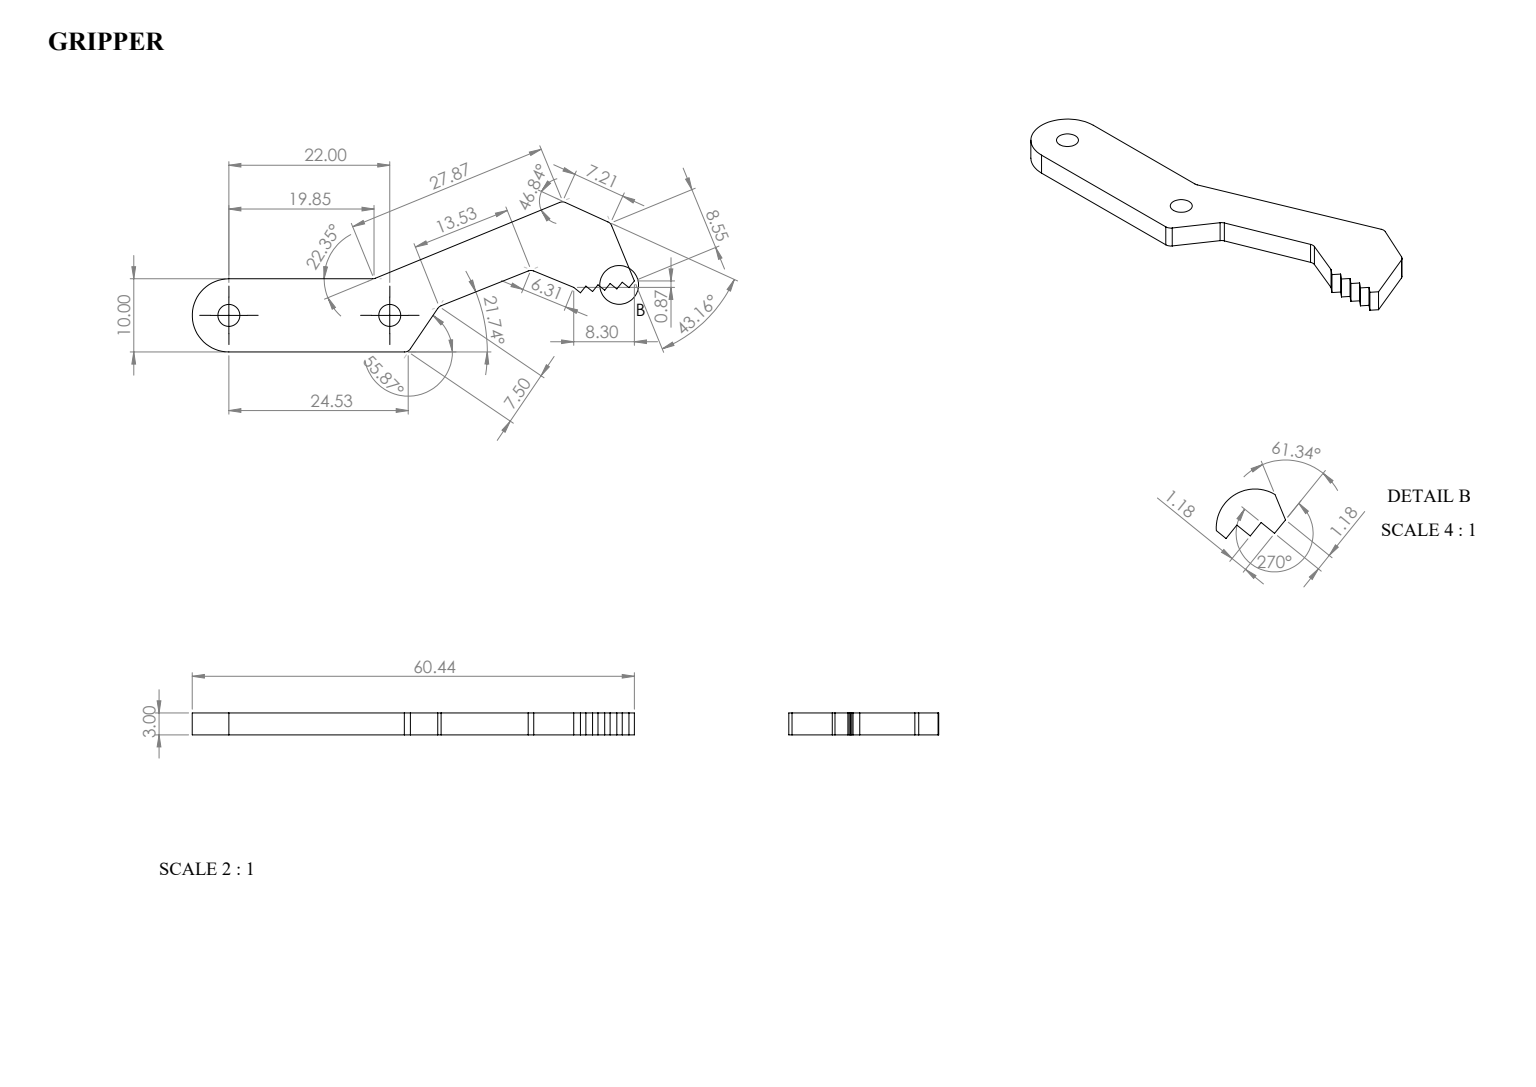
ISO-10303-21;
HEADER;
FILE_DESCRIPTION (('STEP AP214'),
    '1' );
FILE_NAME ('gripper.step',
    '2026-10-11T23:18:24',
    ( '' ),
    ( '' ),
    'SwSTEP 2.0',
    'SolidWorks 2021',
    '' );
FILE_SCHEMA (( 'AUTOMOTIVE_DESIGN' ));
ENDSEC;

DATA;
#11=PLANE ( 'NONE',  #4028 ) ;
#15=CARTESIAN_POINT ( 'NONE',  ( 45.22938609343211880, 3.000000000000000000, -15.43472716196784233 ) ) ;
#33=LINE ( 'NONE', #12635, #7280 ) ;
#53=CARTESIAN_POINT ( 'NONE',  ( 0.000000000000000000, 3.000000000000000000, 0.000000000000000000 ) ) ;
#54=CARTESIAN_POINT ( 'NONE',  ( 41.29994854050690378, 3.000000000000000000, -5.141175130212632283 ) ) ;
#66=AXIS2_PLACEMENT_3D ( 'NONE', #5412, #190, #2837 ) ;
#85=DIRECTION ( 'NONE',  ( 0.7772490812545796990, 0.000000000000000000, 0.6291930273683203900 ) ) ;
#143=DIRECTION ( 'NONE',  ( -0.6291930273683257191, 0.000000000000000000, 0.7772490812545752581 ) ) ;
#190=DIRECTION ( 'NONE',  ( -0.000000000000000000, -1.000000000000000000, -0.000000000000000000 ) ) ;
#201=DIRECTION ( 'NONE',  ( 0.6291930273683254971, 0.000000000000000000, -0.7772490812545754801 ) ) ;
#217=FACE_OUTER_BOUND ( 'NONE', #13506, .T. ) ;
#223=DIRECTION ( 'NONE',  ( -0.000000000000000000, -1.000000000000000000, -0.000000000000000000 ) ) ;
#250=ADVANCED_FACE ( 'NONE', ( #4318 ), #7479, .T. ) ;
#285=AXIS2_PLACEMENT_3D ( 'NONE', #7655, #11797, #366 ) ;
#289=DIRECTION ( 'NONE',  ( 0.7772490812545727046, 0.000000000000000000, 0.6291930273683288277 ) ) ;
#291=VERTEX_POINT ( 'NONE', #13245 ) ;
#292=ORIENTED_EDGE ( 'NONE', *, *, #12896, .T. ) ;
#295=CIRCLE ( 'NONE', #8842, 5.000000000000000000 ) ;
#344=VERTEX_POINT ( 'NONE', #5616 ) ;
#359=ORIENTED_EDGE ( 'NONE', *, *, #9429, .F. ) ;
#362=EDGE_CURVE ( 'NONE', #1968, #1088, #10282, .T. ) ;
#366=DIRECTION ( 'NONE',  ( 0.000000000000000000, 0.000000000000000000, -1.000000000000000000 ) ) ;
#372=ORIENTED_EDGE ( 'NONE', *, *, #1521, .T. ) ;
#388=EDGE_CURVE ( 'NONE', #9987, #6903, #13386, .T. ) ;
#417=ORIENTED_EDGE ( 'NONE', *, *, #1401, .T. ) ;
#424=CARTESIAN_POINT ( 'NONE',  ( 50.46378962010818015, 3.000000000000000000, -4.178819016005276943 ) ) ;
#432=EDGE_CURVE ( 'NONE', #1362, #2254, #9941, .T. ) ;
#437=DIRECTION ( 'NONE',  ( 0.6291930273683107311, 0.000000000000000000, -0.7772490812545873595 ) ) ;
#446=ORIENTED_EDGE ( 'NONE', *, *, #6514, .F. ) ;
#464=VERTEX_POINT ( 'NONE', #3179 ) ;
#465=AXIS2_PLACEMENT_3D ( 'NONE', #7088, #12335, #6953 ) ;
#488=LINE ( 'NONE', #2617, #1153 ) ;
#498=CARTESIAN_POINT ( 'NONE',  ( 0.000000000000000000, 0.000000000000000000, 5.000000000000000000 ) ) ;
#515=CARTESIAN_POINT ( 'NONE',  ( 22.00000000000000000, 0.000000000000000000, 0.000000000000000000 ) ) ;
#530=PLANE ( 'NONE',  #9767 ) ;
#532=CARTESIAN_POINT ( 'NONE',  ( 19.65244806805498357, 3.000000000000000000, -6.000000000000000000 ) ) ;
#534=CARTESIAN_POINT ( 'NONE',  ( 20.03271148078819408, 3.000000000000000000, -5.075121771833452478 ) ) ;
#572=CARTESIAN_POINT ( 'NONE',  ( 52.34174591811297717, 3.000000000000000000, -12.24483450274845531 ) ) ;
#578=VERTEX_POINT ( 'NONE', #7650 ) ;
#584=DIRECTION ( 'NONE',  ( 0.000000000000000000, 1.000000000000000000, 0.000000000000000000 ) ) ;
#587=LINE ( 'NONE', #922, #674 ) ;
#589=FACE_OUTER_BOUND ( 'NONE', #13557, .T. ) ;
#593=CARTESIAN_POINT ( 'NONE',  ( 49.72134184781355515, 0.000000000000000000, -3.261665100124877981 ) ) ;
#596=EDGE_CURVE ( 'NONE', #2976, #3318, #5708, .T. ) ;
#601=DIRECTION ( 'NONE',  ( 0.000000000000000000, 1.000000000000000000, 0.000000000000000000 ) ) ;
#610=ORIENTED_EDGE ( 'NONE', *, *, #4580, .T. ) ;
#641=VERTEX_POINT ( 'NONE', #2277 ) ;
#646=DIRECTION ( 'NONE',  ( -0.7772490812545873595, 0.000000000000000000, -0.6291930273683107311 ) ) ;
#662=AXIS2_PLACEMENT_3D ( 'NONE', #2861, #601, #2728 ) ;
#664=DIRECTION ( 'NONE',  ( 0.9248782281665489657, 0.000000000000000000, -0.3802634127332067404 ) ) ;
#666=EDGE_CURVE ( 'NONE', #1008, #7348, #6486, .T. ) ;
#674=VECTOR ( 'NONE', #7131, 1000.000000000000000 ) ;
#691=ORIENTED_EDGE ( 'NONE', *, *, #2431, .T. ) ;
#702=FACE_OUTER_BOUND ( 'NONE', #12220, .T. ) ;
#728=VECTOR ( 'NONE', #13325, 1000.000000000000000 ) ;
#731=VECTOR ( 'NONE', #11588, 1000.000000000000000 ) ;
#739=CARTESIAN_POINT ( 'NONE',  ( 53.04054522416362261, 3.000000000000000000, -3.611077387296437013 ) ) ;
#770=EDGE_CURVE ( 'NONE', #5898, #6650, #5857, .T. ) ;
#782=CIRCLE ( 'NONE', #5181, 1.500000000000000666 ) ;
#791=MECHANICAL_DESIGN_GEOMETRIC_PRESENTATION_REPRESENTATION('',(#6937),#11784);
#794=CARTESIAN_POINT ( 'NONE',  ( 20.03271148078819408, 0.000000000000000000, -5.075121771833452478 ) ) ;
#795=EDGE_CURVE ( 'NONE', #291, #13143, #3919, .T. ) ;
#799=CARTESIAN_POINT ( 'NONE',  ( 48.80418793193314997, 0.000000000000000000, -4.004112872419501201 ) ) ;
#814=DIRECTION ( 'NONE',  ( -0.4145344181384821858, 0.000000000000000000, 0.9100336346413741007 ) ) ;
#826=LINE ( 'NONE', #5339, #12157 ) ;
#830=ORIENTED_EDGE ( 'NONE', *, *, #11288, .T. ) ;
#835=( LENGTH_UNIT ( ) NAMED_UNIT ( * ) SI_UNIT ( .MILLI., .METRE. ) );
#847=ORIENTED_EDGE ( 'NONE', *, *, #2780, .F. ) ;
#860=EDGE_CURVE ( 'NONE', #10776, #641, #1589, .T. ) ;
#876=CARTESIAN_POINT ( 'NONE',  ( 29.02231267299996986, 3.000000000000000000, -1.321950885510182250 ) ) ;
#885=EDGE_CURVE ( 'NONE', #12346, #7762, #8457, .T. ) ;
#922=CARTESIAN_POINT ( 'NONE',  ( 48.80418793193314997, 3.000000000000000000, -4.004112872419501201 ) ) ;
#925=FACE_OUTER_BOUND ( 'NONE', #3987, .T. ) ;
#944=LINE ( 'NONE', #5143, #12861 ) ;
#967=ORIENTED_EDGE ( 'NONE', *, *, #13406, .T. ) ;
#977=DIRECTION ( 'NONE',  ( 0.7772490812545771455, 0.000000000000000000, 0.6291930273683233876 ) ) ;
#1007=VECTOR ( 'NONE', #3151, 1000.000000000000000 ) ;
#1008=VERTEX_POINT ( 'NONE', #7434 ) ;
#1037=DIRECTION ( 'NONE',  ( -0.7772490812545750360, 0.000000000000000000, -0.6291930273683260522 ) ) ;
#1041=EDGE_CURVE ( 'NONE', #6903, #7175, #2191, .T. ) ;
#1052=FACE_OUTER_BOUND ( 'NONE', #12922, .T. ) ;
#1074=DIRECTION ( 'NONE',  ( -0.000000000000000000, -1.000000000000000000, -0.000000000000000000 ) ) ;
#1075=ORIENTED_EDGE ( 'NONE', *, *, #12735, .T. ) ;
#1088=VERTEX_POINT ( 'NONE', #8584 ) ;
#1107=ORIENTED_EDGE ( 'NONE', *, *, #3844, .F. ) ;
#1113=ORIENTED_EDGE ( 'NONE', *, *, #9512, .F. ) ;
#1127=ORIENTED_EDGE ( 'NONE', *, *, #9053, .T. ) ;
#1150=DIRECTION ( 'NONE',  ( 0.7772490812545826966, 0.000000000000000000, 0.6291930273683166153 ) ) ;
#1153=VECTOR ( 'NONE', #7917, 1000.000000000000000 ) ;
#1160=ORIENTED_EDGE ( 'NONE', *, *, #11475, .F. ) ;
#1161=AXIS2_PLACEMENT_3D ( 'NONE', #2598, #10999, #1573 ) ;
#1187=ORIENTED_EDGE ( 'NONE', *, *, #8298, .F. ) ;
#1210=AXIS2_PLACEMENT_3D ( 'NONE', #424, #12838, #1323 ) ;
#1222=ORIENTED_EDGE ( 'NONE', *, *, #12916, .F. ) ;
#1226=DIRECTION ( 'NONE',  ( 0.6291930273683290498, 0.000000000000000000, -0.7772490812545727046 ) ) ;
#1244=CARTESIAN_POINT ( 'NONE',  ( 23.99887587215152607, 3.000000000000000000, 4.000000000000000000 ) ) ;
#1250=CARTESIAN_POINT ( 'NONE',  ( 19.65244806805498001, 3.000000000000000000, -5.000000000000000000 ) ) ;
#1264=ORIENTED_EDGE ( 'NONE', *, *, #2886, .T. ) ;
#1265=ORIENTED_EDGE ( 'NONE', *, *, #666, .F. ) ;
#1281=LINE ( 'NONE', #10781, #3594 ) ;
#1294=ORIENTED_EDGE ( 'NONE', *, *, #11288, .F. ) ;
#1297=ADVANCED_FACE ( 'NONE', ( #5972 ), #12048, .F. ) ;
#1311=ORIENTED_EDGE ( 'NONE', *, *, #885, .F. ) ;
#1313=ORIENTED_EDGE ( 'NONE', *, *, #10118, .T. ) ;
#1323=DIRECTION ( 'NONE',  ( -0.7772490812545771455, 0.000000000000000000, -0.6291930273683233876 ) ) ;
#1325=DIRECTION ( 'NONE',  ( -0.9288742131985401329, 0.000000000000000000, 0.3703953240185315909 ) ) ;
#1342=EDGE_CURVE ( 'NONE', #7762, #9987, #8243, .T. ) ;
#1348=DIRECTION ( 'NONE',  ( 0.5610724890695777400, 0.000000000000000000, -0.8277666712360848278 ) ) ;
#1352=DIRECTION ( 'NONE',  ( 0.6291930273683254971, 0.000000000000000000, -0.7772490812545754801 ) ) ;
#1362=VERTEX_POINT ( 'NONE', #4171 ) ;
#1373=DIRECTION ( 'NONE',  ( 0.000000000000000000, 1.000000000000000000, 0.000000000000000000 ) ) ;
#1383=VERTEX_POINT ( 'NONE', #6116 ) ;
#1401=EDGE_CURVE ( 'NONE', #12205, #5887, #5126, .T. ) ;
#1404=VECTOR ( 'NONE', #9043, 1000.000000000000000 ) ;
#1411=CARTESIAN_POINT ( 'NONE',  ( 0.000000000000000000, 3.000000000000000000, 0.000000000000000000 ) ) ;
#1419=VERTEX_POINT ( 'NONE', #4785 ) ;
#1443=AXIS2_PLACEMENT_3D ( 'NONE', #11916, #10885, #1450 ) ;
#1445=EDGE_CURVE ( 'NONE', #11616, #8766, #4718, .T. ) ;
#1450=DIRECTION ( 'NONE',  ( 0.000000000000000000, 0.000000000000000000, -1.000000000000000000 ) ) ;
#1475=CARTESIAN_POINT ( 'NONE',  ( 47.14458624375820506, 0.000000000000000000, -3.829406728833672613 ) ) ;
#1511=CARTESIAN_POINT ( 'NONE',  ( 29.39270799701850123, 3.000000000000000000, -0.3930766723116408401 ) ) ;
#1521=EDGE_CURVE ( 'NONE', #3318, #464, #2714, .T. ) ;
#1564=CARTESIAN_POINT ( 'NONE',  ( 22.00000000000000000, 3.000000000000000000, -1.500000000000000666 ) ) ;
#1569=EDGE_CURVE ( 'NONE', #5437, #5898, #5276, .T. ) ;
#1573=DIRECTION ( 'NONE',  ( -1.000000000000000000, 0.000000000000000000, -0.000000000000000000 ) ) ;
#1589=LINE ( 'NONE', #3857, #4670 ) ;
#1592=VERTEX_POINT ( 'NONE', #12597 ) ;
#1605=PRODUCT_DEFINITION ( 'UNKNOWN', '', #8267, #12345 ) ;
#1606=FACE_OUTER_BOUND ( 'NONE', #1630, .T. ) ;
#1628=EDGE_LOOP ( 'NONE', ( #967, #8471, #2768, #4879 ) ) ;
#1630=EDGE_LOOP ( 'NONE', ( #9979, #6504, #3840, #12459, #9427, #11054, #12260, #11882, #1794, #1294, #6593, #5923, #12223, #9618, #6732, #1311, #5467, #13454, #10169, #1160, #8458, #5363, #5414, #7618, #8830, #3725, #12842 ) ) ;
#1636=CARTESIAN_POINT ( 'NONE',  ( 45.60964950616533287, 0.000000000000000000, -14.50984893380129392 ) ) ;
#1637=FACE_OUTER_BOUND ( 'NONE', #7799, .T. ) ;
#1665=CARTESIAN_POINT ( 'NONE',  ( 54.70014691233865989, 3.000000000000000000, -3.785783530882224746 ) ) ;
#1671=DIRECTION ( 'NONE',  ( -0.7772490812546181127, 0.000000000000000000, -0.6291930273682727615 ) ) ;
#1683=ORIENTED_EDGE ( 'NONE', *, *, #770, .T. ) ;
#1724=DIRECTION ( 'NONE',  ( 0.000000000000000000, 0.000000000000000000, -1.000000000000000000 ) ) ;
#1733=EDGE_CURVE ( 'NONE', #8766, #12346, #10724, .T. ) ;
#1738=FACE_OUTER_BOUND ( 'NONE', #5719, .T. ) ;
#1770=VECTOR ( 'NONE', #4286, 1000.000000000000000 ) ;
#1773=EDGE_CURVE ( 'NONE', #3986, #6650, #1281, .T. ) ;
#1780=CIRCLE ( 'NONE', #9471, 1.000000000000000888 ) ;
#1781=ORIENTED_EDGE ( 'NONE', *, *, #2886, .F. ) ;
#1788=EDGE_CURVE ( 'NONE', #2335, #10776, #7481, .T. ) ;
#1794=ORIENTED_EDGE ( 'NONE', *, *, #13063, .F. ) ;
#1804=CARTESIAN_POINT ( 'NONE',  ( 22.00000000000000000, 3.000000000000000000, -1.500000000000000666 ) ) ;
#1840=DIRECTION ( 'NONE',  ( 0.000000000000000000, 0.000000000000000000, -1.000000000000000000 ) ) ;
#1850=VECTOR ( 'NONE', #1150, 1000.000000000000227 ) ;
#1863=DIRECTION ( 'NONE',  ( -0.000000000000000000, -1.000000000000000000, -0.000000000000000000 ) ) ;
#1867=ORIENTED_EDGE ( 'NONE', *, *, #432, .T. ) ;
#1877=SURFACE_SIDE_STYLE ('',( #11233 ) ) ;
#1901=EDGE_CURVE ( 'NONE', #6718, #12346, #8914, .T. ) ;
#1918=CYLINDRICAL_SURFACE ( 'NONE', #5087, 1.000000000000000888 ) ;
#1942=DIRECTION ( 'NONE',  ( -0.000000000000000000, -1.000000000000000000, -0.000000000000000000 ) ) ;
#1962=ORIENTED_EDGE ( 'NONE', *, *, #388, .T. ) ;
#1968=VERTEX_POINT ( 'NONE', #6164 ) ;
#1973=CARTESIAN_POINT ( 'NONE',  ( 55.44259468463320673, 3.000000000000000000, -4.702937446762657459 ) ) ;
#1996=ORIENTED_EDGE ( 'NONE', *, *, #12521, .F. ) ;
#2009=LINE ( 'NONE', #6271, #5183 ) ;
#2019=DIRECTION ( 'NONE',  ( 0.000000000000000000, 0.000000000000000000, 1.000000000000000000 ) ) ;
#2026=AXIS2_PLACEMENT_3D ( 'NONE', #8392, #1373, #7643 ) ;
#2035=VECTOR ( 'NONE', #4236, 1000.000000000000000 ) ;
#2052=CARTESIAN_POINT ( 'NONE',  ( 24.82664254338761722, 3.000000000000000000, 4.561072489069574409 ) ) ;
#2058=DIRECTION ( 'NONE',  ( -0.000000000000000000, -1.000000000000000000, -0.000000000000000000 ) ) ;
#2061=DIRECTION ( 'NONE',  ( -0.000000000000000000, -1.000000000000000000, -0.000000000000000000 ) ) ;
#2082=VERTEX_POINT ( 'NONE', #11267 ) ;
#2085=DIRECTION ( 'NONE',  ( 0.000000000000000000, 0.000000000000000000, -1.000000000000000000 ) ) ;
#2088=DIRECTION ( 'NONE',  ( 0.000000000000000000, 0.000000000000000000, -1.000000000000000000 ) ) ;
#2099=VERTEX_POINT ( 'NONE', #10241 ) ;
#2102=ORIENTED_EDGE ( 'NONE', *, *, #8983, .T. ) ;
#2144=ORIENTED_EDGE ( 'NONE', *, *, #7522, .T. ) ;
#2169=DIRECTION ( 'NONE',  ( 0.6291930273683260522, 0.000000000000000000, -0.7772490812545749250 ) ) ;
#2171=PLANE ( 'NONE',  #12135 ) ;
#2187=LINE ( 'NONE', #11973, #6238 ) ;
#2191=LINE ( 'NONE', #13571, #2255 ) ;
#2203=ORIENTED_EDGE ( 'NONE', *, *, #4595, .T. ) ;
#2216=CARTESIAN_POINT ( 'NONE',  ( 53.78299299645824050, 3.000000000000000000, -4.528231303176834643 ) ) ;
#2239=VERTEX_POINT ( 'NONE', #10842 ) ;
#2246=CIRCLE ( 'NONE', #285, 1.000000000000000000 ) ;
#2247=AXIS2_PLACEMENT_3D ( 'NONE', #12014, #2569, #13172 ) ;
#2248=CARTESIAN_POINT ( 'NONE',  ( 47.14458624375820506, 3.000000000000000000, -3.829406728833672613 ) ) ;
#2254=VERTEX_POINT ( 'NONE', #7933 ) ;
#2255=VECTOR ( 'NONE', #6389, 1000.000000000000000 ) ;
#2268=VECTOR ( 'NONE', #13335, 1000.000000000000000 ) ;
#2277=CARTESIAN_POINT ( 'NONE',  ( 48.80418793193314997, 0.000000000000000000, -4.004112872419501201 ) ) ;
#2278=EDGE_CURVE ( 'NONE', #2254, #7268, #10593, .T. ) ;
#2293=CARTESIAN_POINT ( 'NONE',  ( 0.000000000000000000, 3.000000000000000000, 5.000000000000000000 ) ) ;
#2299=ORIENTED_EDGE ( 'NONE', *, *, #795, .T. ) ;
#2312=PLANE ( 'NONE',  #8209 ) ;
#2335=VERTEX_POINT ( 'NONE', #1475 ) ;
#2336=PRODUCT_CONTEXT ( 'NONE', #3509, 'mechanical' ) ;
#2385=CARTESIAN_POINT ( 'NONE',  ( 52.12339130828321032, 0.000000000000000000, -4.353525159591052685 ) ) ;
#2388=EDGE_CURVE ( 'NONE', #11595, #10663, #6143, .T. ) ;
#2392=CARTESIAN_POINT ( 'NONE',  ( 41.67875868938293138, 0.000000000000000000, -6.066649533482935119 ) ) ;
#2395=ORIENTED_EDGE ( 'NONE', *, *, #8983, .F. ) ;
#2431=EDGE_CURVE ( 'NONE', #4566, #7781, #13590, .T. ) ;
#2458=DIRECTION ( 'NONE',  ( 0.9254744032703045020, 0.000000000000000000, 0.3788101488760216018 ) ) ;
#2476=CYLINDRICAL_SURFACE ( 'NONE', #4736, 1.000000000000000444 ) ;
#2505=ORIENTED_EDGE ( 'NONE', *, *, #13043, .F. ) ;
#2518=CIRCLE ( 'NONE', #8237, 1.500000000000000222 ) ;
#2520=VECTOR ( 'NONE', #3875, 1000.000000000000000 ) ;
#2524=DIRECTION ( 'NONE',  ( 0.000000000000000000, 0.000000000000000000, 1.000000000000000000 ) ) ;
#2531=DIRECTION ( 'NONE',  ( -0.000000000000000000, -1.000000000000000000, -0.000000000000000000 ) ) ;
#2533=EDGE_LOOP ( 'NONE', ( #3440, #12296, #7097, #7171 ) ) ;
#2551=LINE ( 'NONE', #8373, #7050 ) ;
#2568=EDGE_LOOP ( 'NONE', ( #11980, #11539, #3859, #1127 ) ) ;
#2569=DIRECTION ( 'NONE',  ( 0.000000000000000000, -1.000000000000000000, 0.000000000000000000 ) ) ;
#2575=PLANE ( 'NONE',  #10618 ) ;
#2598=CARTESIAN_POINT ( 'NONE',  ( 0.000000000000000000, 3.000000000000000000, 5.000000000000000000 ) ) ;
#2617=CARTESIAN_POINT ( 'NONE',  ( 45.60964950616533287, 3.000000000000000000, -15.50984893380129392 ) ) ;
#2622=LINE ( 'NONE', #3865, #12146 ) ;
#2649=DIRECTION ( 'NONE',  ( 0.000000000000000000, 0.000000000000000000, -1.000000000000000000 ) ) ;
#2691=DIRECTION ( 'NONE',  ( -0.9100336346413742117, -0.000000000000000000, -0.4145344181384821858 ) ) ;
#2694=FACE_BOUND ( 'NONE', #2698, .T. ) ;
#2698=EDGE_LOOP ( 'NONE', ( #8476, #417 ) ) ;
#2700=ORIENTED_EDGE ( 'NONE', *, *, #7210, .T. ) ;
#2714=LINE ( 'NONE', #11189, #4255 ) ;
#2728=DIRECTION ( 'NONE',  ( 0.000000000000000000, 0.000000000000000000, 1.000000000000000000 ) ) ;
#2751=CARTESIAN_POINT ( 'NONE',  ( 53.04054522416362261, 0.000000000000000000, -3.611077387296437013 ) ) ;
#2759=EDGE_LOOP ( 'NONE', ( #4791, #11244, #3057, #10602 ) ) ;
#2768=ORIENTED_EDGE ( 'NONE', *, *, #4568, .F. ) ;
#2780=EDGE_CURVE ( 'NONE', #13316, #10663, #7108, .T. ) ;
#2784=CARTESIAN_POINT ( 'NONE',  ( 29.02231267299996986, 3.000000000000000000, -1.321950885510182250 ) ) ;
#2787=ORIENTED_EDGE ( 'NONE', *, *, #9935, .F. ) ;
#2792=DIRECTION ( 'NONE',  ( 0.000000000000000000, 1.000000000000000000, -0.000000000000000000 ) ) ;
#2803=EDGE_LOOP ( 'NONE', ( #5343, #13058, #2787, #6487 ) ) ;
#2804=ORIENTED_EDGE ( 'NONE', *, *, #12721, .F. ) ;
#2811=DIRECTION ( 'NONE',  ( 0.000000000000000000, 1.000000000000000000, -0.000000000000000000 ) ) ;
#2826=CARTESIAN_POINT ( 'NONE',  ( 51.41686768994642165, 3.000000000000000000, -11.86457109001525545 ) ) ;
#2837=DIRECTION ( 'NONE',  ( 0.000000000000000000, 0.000000000000000000, -1.000000000000000000 ) ) ;
#2849=DIRECTION ( 'NONE',  ( 0.6291930273682743158, 0.000000000000000000, -0.7772490812546168915 ) ) ;
#2861=CARTESIAN_POINT ( 'NONE',  ( 22.00000000000000000, 3.000000000000000000, 0.000000000000000000 ) ) ;
#2864=PLANE ( 'NONE',  #6038 ) ;
#2865=CARTESIAN_POINT ( 'NONE',  ( 24.82664254338761722, 3.000000000000000000, 4.561072489069574409 ) ) ;
#2880=CIRCLE ( 'NONE', #10802, 1.500000000000000666 ) ;
#2882=AXIS2_PLACEMENT_3D ( 'NONE', #2248, #1226, #11762 ) ;
#2886=EDGE_CURVE ( 'NONE', #2239, #2099, #3058, .T. ) ;
#2892=EDGE_CURVE ( 'NONE', #6179, #5887, #11232, .T. ) ;
#2913=VECTOR ( 'NONE', #11160, 1000.000000000000000 ) ;
#2923=CARTESIAN_POINT ( 'NONE',  ( 52.12339130828321032, 3.000000000000000000, -4.353525159591052685 ) ) ;
#2938=DIRECTION ( 'NONE',  ( 0.000000000000000000, 0.000000000000000000, -1.000000000000000000 ) ) ;
#2970=CARTESIAN_POINT ( 'NONE',  ( 53.04054522416362261, 3.000000000000000000, -3.611077387296437013 ) ) ;
#2976=VERTEX_POINT ( 'NONE', #3286 ) ;
#3050=DIRECTION ( 'NONE',  ( -0.000000000000000000, -1.000000000000000000, -0.000000000000000000 ) ) ;
#3053=ORIENTED_EDGE ( 'NONE', *, *, #3579, .T. ) ;
#3055=ORIENTED_EDGE ( 'NONE', *, *, #596, .T. ) ;
#3057=ORIENTED_EDGE ( 'NONE', *, *, #1569, .F. ) ;
#3058=CIRCLE ( 'NONE', #8763, 0.9999999999999991118 ) ;
#3079=DIRECTION ( 'NONE',  ( 0.000000000000000000, 0.000000000000000000, 1.000000000000000000 ) ) ;
#3091=VECTOR ( 'NONE', #3849, 1000.000000000000114 ) ;
#3101=EDGE_LOOP ( 'NONE', ( #12387, #11429 ) ) ;
#3102=ORIENTED_EDGE ( 'NONE', *, *, #6600, .T. ) ;
#3120=ADVANCED_FACE ( 'NONE', ( #3564, #11005, #6676 ), #12050, .F. ) ;
#3129=CARTESIAN_POINT ( 'NONE',  ( 0.000000000000000000, 3.000000000000000000, -1.500000000000000222 ) ) ;
#3151=DIRECTION ( 'NONE',  ( -0.000000000000000000, -1.000000000000000000, -0.000000000000000000 ) ) ;
#3173=PLANE ( 'NONE',  #6883 ) ;
#3179=CARTESIAN_POINT ( 'NONE',  ( 48.80418793193314997, 3.000000000000000000, -4.004112872419501201 ) ) ;
#3217=EDGE_CURVE ( 'NONE', #5437, #3986, #13288, .T. ) ;
#3222=ORIENTED_EDGE ( 'NONE', *, *, #795, .F. ) ;
#3239=ORIENTED_EDGE ( 'NONE', *, *, #1342, .T. ) ;
#3286=CARTESIAN_POINT ( 'NONE',  ( 47.14458624375820506, 3.000000000000000000, -3.829406728833672613 ) ) ;
#3293=CARTESIAN_POINT ( 'NONE',  ( 41.67875868938293138, 0.000000000000000000, -6.066649533482935119 ) ) ;
#3318=VERTEX_POINT ( 'NONE', #4115 ) ;
#3333=ORIENTED_EDGE ( 'NONE', *, *, #13043, .T. ) ;
#3365=AXIS2_PLACEMENT_3D ( 'NONE', #7869, #9118, #12090 ) ;
#3369=DIRECTION ( 'NONE',  ( -0.000000000000000000, -1.000000000000000000, -0.000000000000000000 ) ) ;
#3381=DIRECTION ( 'NONE',  ( 0.000000000000000000, 0.000000000000000000, 1.000000000000000000 ) ) ;
#3429=DIRECTION ( 'NONE',  ( 0.000000000000000000, 0.000000000000000000, -1.000000000000000000 ) ) ;
#3440=ORIENTED_EDGE ( 'NONE', *, *, #1788, .T. ) ;
#3447=LINE ( 'NONE', #2216, #8622 ) ;
#3453=FACE_OUTER_BOUND ( 'NONE', #2568, .T. ) ;
#3473=EDGE_CURVE ( 'NONE', #10535, #2976, #2551, .T. ) ;
#3509=APPLICATION_CONTEXT ( 'automotive_design' ) ;
#3546=LINE ( 'NONE', #6657, #12791 ) ;
#3564=FACE_OUTER_BOUND ( 'NONE', #5744, .T. ) ;
#3579=EDGE_CURVE ( 'NONE', #2082, #13415, #3666, .T. ) ;
#3592=PLANE ( 'NONE',  #2247 ) ;
#3594=VECTOR ( 'NONE', #1348, 1000.000000000000000 ) ;
#3641=ORIENTED_EDGE ( 'NONE', *, *, #13521, .T. ) ;
#3656=FACE_BOUND ( 'NONE', #5012, .T. ) ;
#3657=EDGE_CURVE ( 'NONE', #12875, #1362, #8214, .T. ) ;
#3660=ORIENTED_EDGE ( 'NONE', *, *, #6391, .T. ) ;
#3666=LINE ( 'NONE', #4841, #5489 ) ;
#3671=DIRECTION ( 'NONE',  ( 0.9288742131985401329, 0.000000000000000000, -0.3703953240185316464 ) ) ;
#3679=CARTESIAN_POINT ( 'NONE',  ( 41.29994854050690378, 3.000000000000000000, -5.141175130212632283 ) ) ;
#3680=CARTESIAN_POINT ( 'NONE',  ( 20.03271148078819408, 3.000000000000000000, -5.075121771833452478 ) ) ;
#3709=EDGE_LOOP ( 'NONE', ( #13077, #1222, #9830, #691 ) ) ;
#3712=( NAMED_UNIT ( * ) PLANE_ANGLE_UNIT ( ) SI_UNIT ( $, .RADIAN. ) );
#3725=ORIENTED_EDGE ( 'NONE', *, *, #432, .F. ) ;
#3734=DIRECTION ( 'NONE',  ( -0.7772490812545826966, 0.000000000000000000, -0.6291930273683166153 ) ) ;
#3772=DIRECTION ( 'NONE',  ( -0.000000000000000000, -1.000000000000000000, 0.000000000000000000 ) ) ;
#3777=UNCERTAINTY_MEASURE_WITH_UNIT (LENGTH_MEASURE( 1.000000000000000082E-05 ), #12389, 'distance_accuracy_value', 'NONE');
#3786=CARTESIAN_POINT ( 'NONE',  ( 51.38094353598858532, 3.000000000000000000, -3.436371243710653722 ) ) ;
#3787=PLANE ( 'NONE',  #10165 ) ;
#3789=VECTOR ( 'NONE', #6193, 1000.000000000000227 ) ;
#3840=ORIENTED_EDGE ( 'NONE', *, *, #5536, .F. ) ;
#3844=EDGE_CURVE ( 'NONE', #1008, #1968, #11860, .T. ) ;
#3849=DIRECTION ( 'NONE',  ( 0.9288742131985401329, 0.000000000000000000, -0.3703953240185316464 ) ) ;
#3857=CARTESIAN_POINT ( 'NONE',  ( 48.06174015963858892, 0.000000000000000000, -3.086958956539055166 ) ) ;
#3859=ORIENTED_EDGE ( 'NONE', *, *, #6600, .F. ) ;
#3865=CARTESIAN_POINT ( 'NONE',  ( 46.02418392430381999, 3.000000000000000000, -15.41988256844266658 ) ) ;
#3875=DIRECTION ( 'NONE',  ( -0.000000000000000000, -1.000000000000000000, -0.000000000000000000 ) ) ;
#3897=DIRECTION ( 'NONE',  ( -0.000000000000000000, -1.000000000000000000, -0.000000000000000000 ) ) ;
#3899=EDGE_CURVE ( 'NONE', #291, #9987, #33, .T. ) ;
#3903=ORIENTED_EDGE ( 'NONE', *, *, #7030, .T. ) ;
#3919=LINE ( 'NONE', #1665, #5113 ) ;
#3933=CARTESIAN_POINT ( 'NONE',  ( 54.70014691233865989, 0.000000000000000000, -3.785783530882224746 ) ) ;
#3963=VECTOR ( 'NONE', #85, 1000.000000000000000 ) ;
#3964=DIRECTION ( 'NONE',  ( -0.000000000000000000, -1.000000000000000000, -0.000000000000000000 ) ) ;
#3971=AXIS2_PLACEMENT_3D ( 'NONE', #11570, #9560, #5477 ) ;
#3977=FACE_OUTER_BOUND ( 'NONE', #3709, .T. ) ;
#3980=AXIS2_PLACEMENT_3D ( 'NONE', #54, #8234, #2938 ) ;
#3983=CIRCLE ( 'NONE', #6188, 1.500000000000000222 ) ;
#3986=VERTEX_POINT ( 'NONE', #12961 ) ;
#3987=EDGE_LOOP ( 'NONE', ( #11228, #3641, #5133, #6699 ) ) ;
#3991=CIRCLE ( 'NONE', #11480, 1.500000000000000222 ) ;
#4023=ORIENTED_EDGE ( 'NONE', *, *, #8102, .F. ) ;
#4027=ORIENTED_EDGE ( 'NONE', *, *, #5513, .T. ) ;
#4028=AXIS2_PLACEMENT_3D ( 'NONE', #2970, #1037, #7035 ) ;
#4053=AXIS2_PLACEMENT_3D ( 'NONE', #12272, #2811, #4605 ) ;
#4057=CARTESIAN_POINT ( 'NONE',  ( 29.02231267299996986, 3.000000000000000000, -1.321950885510182250 ) ) ;
#4059=UNCERTAINTY_MEASURE_WITH_UNIT (LENGTH_MEASURE( 1.000000000000000082E-05 ), #5864, 'distance_accuracy_value', 'NONE');
#4080=EDGE_LOOP ( 'NONE', ( #12049, #4926, #1107, #10377 ) ) ;
#4093=LINE ( 'NONE', #2923, #7517 ) ;
#4106=LINE ( 'NONE', #3129, #9476 ) ;
#4115=CARTESIAN_POINT ( 'NONE',  ( 48.06174015963858892, 3.000000000000000000, -3.086958956539055166 ) ) ;
#4136=CARTESIAN_POINT ( 'NONE',  ( 22.00000000000000000, 0.000000000000000000, 1.500000000000000666 ) ) ;
#4144=EDGE_CURVE ( 'NONE', #11098, #578, #1780, .T. ) ;
#4171=CARTESIAN_POINT ( 'NONE',  ( 40.92955321648837241, 0.000000000000000000, -6.070049343411170639 ) ) ;
#4172=EDGE_CURVE ( 'NONE', #464, #4566, #7379, .T. ) ;
#4187=ORIENTED_EDGE ( 'NONE', *, *, #12187, .T. ) ;
#4214=VECTOR ( 'NONE', #10335, 1000.000000000000227 ) ;
#4233=DIRECTION ( 'NONE',  ( 0.000000000000000000, 1.000000000000000000, 0.000000000000000000 ) ) ;
#4234=FACE_OUTER_BOUND ( 'NONE', #5627, .T. ) ;
#4236=DIRECTION ( 'NONE',  ( -0.000000000000000000, -1.000000000000000000, -0.000000000000000000 ) ) ;
#4255=VECTOR ( 'NONE', #2849, 1000.000000000000000 ) ;
#4260=ORIENTED_EDGE ( 'NONE', *, *, #4172, .F. ) ;
#4278=MECHANICAL_DESIGN_GEOMETRIC_PRESENTATION_REPRESENTATION('',(#12869),#7584);
#4286=DIRECTION ( 'NONE',  ( -1.000000000000000000, -0.000000000000000000, -0.000000000000000000 ) ) ;
#4318=FACE_OUTER_BOUND ( 'NONE', #8137, .T. ) ;
#4354=DIRECTION ( 'NONE',  ( 0.000000000000000000, 1.000000000000000000, 0.000000000000000000 ) ) ;
#4383=DIRECTION ( 'NONE',  ( 0.000000000000000000, 1.000000000000000000, 0.000000000000000000 ) ) ;
#4387=CARTESIAN_POINT ( 'NONE',  ( 47.14458624375820506, 3.000000000000000000, -3.829406728833672613 ) ) ;
#4403=AXIS2_PLACEMENT_3D ( 'NONE', #11454, #8084, #10427 ) ;
#4424=EDGE_LOOP ( 'NONE', ( #7431, #7570, #10921, #12591 ) ) ;
#4430=ADVANCED_FACE ( 'NONE', ( #3977 ), #11215, .F. ) ;
#4460=ORIENTED_EDGE ( 'NONE', *, *, #3473, .T. ) ;
#4501=ADVANCED_FACE ( 'NONE', ( #5979 ), #5281, .F. ) ;
#4521=DIRECTION ( 'NONE',  ( 0.7772490812545727046, 0.000000000000000000, 0.6291930273683288277 ) ) ;
#4566=VERTEX_POINT ( 'NONE', #11490 ) ;
#4568=EDGE_CURVE ( 'NONE', #5777, #9675, #11903, .T. ) ;
#4580=EDGE_CURVE ( 'NONE', #13415, #7348, #9904, .T. ) ;
#4595=EDGE_CURVE ( 'NONE', #7175, #10532, #5298, .T. ) ;
#4603=DIRECTION ( 'NONE',  ( 0.000000000000000000, -1.000000000000000000, 0.000000000000000000 ) ) ;
#4605=DIRECTION ( 'NONE',  ( 0.000000000000000000, 0.000000000000000000, -1.000000000000000000 ) ) ;
#4607=CYLINDRICAL_SURFACE ( 'NONE', #1443, 0.9999999999999991118 ) ;
#4652=CYLINDRICAL_SURFACE ( 'NONE', #7572, 1.000000000000000888 ) ;
#4670=VECTOR ( 'NONE', #5919, 1000.000000000000000 ) ;
#4717=DIRECTION ( 'NONE',  ( 0.000000000000000000, 1.000000000000000000, 0.000000000000000000 ) ) ;
#4718=LINE ( 'NONE', #10232, #1404 ) ;
#4735=CARTESIAN_POINT ( 'NONE',  ( 46.02418392430381999, 0.000000000000000000, -15.41988256844266836 ) ) ;
#4736=AXIS2_PLACEMENT_3D ( 'NONE', #1244, #3369, #10745 ) ;
#4739=ORIENTED_EDGE ( 'NONE', *, *, #13063, .T. ) ;
#4743=EDGE_CURVE ( 'NONE', #4566, #1383, #3546, .T. ) ;
#4779=DIRECTION ( 'NONE',  ( 0.000000000000000000, 0.000000000000000000, 1.000000000000000000 ) ) ;
#4785=CARTESIAN_POINT ( 'NONE',  ( 29.02231267299996986, 0.000000000000000000, -1.321950885510182250 ) ) ;
#4789=EDGE_CURVE ( 'NONE', #13316, #11616, #4859, .T. ) ;
#4791=ORIENTED_EDGE ( 'NONE', *, *, #1773, .T. ) ;
#4798=DIRECTION ( 'NONE',  ( 0.000000000000000000, 1.000000000000000000, 0.000000000000000000 ) ) ;
#4800=DIRECTION ( 'NONE',  ( -0.000000000000000000, -1.000000000000000000, -0.000000000000000000 ) ) ;
#4810=CARTESIAN_POINT ( 'NONE',  ( 29.39270799701850123, 0.000000000000000000, -0.3930766723116408401 ) ) ;
#4817=EDGE_CURVE ( 'NONE', #6179, #12863, #8590, .T. ) ;
#4841=CARTESIAN_POINT ( 'NONE',  ( 20.03271148078819408, 3.000000000000000000, -5.075121771833452478 ) ) ;
#4859=LINE ( 'NONE', #6935, #6806 ) ;
#4860=FACE_OUTER_BOUND ( 'NONE', #2803, .T. ) ;
#4879=ORIENTED_EDGE ( 'NONE', *, *, #6391, .F. ) ;
#4907=EDGE_LOOP ( 'NONE', ( #7267, #10315, #4739, #12364 ) ) ;
#4926=ORIENTED_EDGE ( 'NONE', *, *, #362, .F. ) ;
#4933=VECTOR ( 'NONE', #7075, 1000.000000000000000 ) ;
#4990=CARTESIAN_POINT ( 'NONE',  ( 53.04054522416362261, 3.000000000000000000, -3.611077387296437013 ) ) ;
#5005=EDGE_CURVE ( 'NONE', #13346, #11587, #3983, .T. ) ;
#5008=PLANE ( 'NONE',  #7556 ) ;
#5012=EDGE_LOOP ( 'NONE', ( #10920, #8741 ) ) ;
#5029=FACE_OUTER_BOUND ( 'NONE', #7031, .T. ) ;
#5059=ORIENTED_EDGE ( 'NONE', *, *, #9844, .T. ) ;
#5071=LINE ( 'NONE', #5966, #4933 ) ;
#5072=DIRECTION ( 'NONE',  ( -0.000000000000000000, -1.000000000000000000, -0.000000000000000000 ) ) ;
#5087=AXIS2_PLACEMENT_3D ( 'NONE', #6170, #5142, #11552 ) ;
#5113=VECTOR ( 'NONE', #11227, 1000.000000000000000 ) ;
#5120=DIRECTION ( 'NONE',  ( -0.000000000000000000, -1.000000000000000000, -0.000000000000000000 ) ) ;
#5126=CIRCLE ( 'NONE', #12617, 1.500000000000000666 ) ;
#5129=VECTOR ( 'NONE', #9308, 1000.000000000000000 ) ;
#5133=ORIENTED_EDGE ( 'NONE', *, *, #2892, .T. ) ;
#5142=DIRECTION ( 'NONE',  ( -0.000000000000000000, -1.000000000000000000, -0.000000000000000000 ) ) ;
#5143=CARTESIAN_POINT ( 'NONE',  ( 50.46378962010818015, 3.000000000000000000, -4.178819016005276943 ) ) ;
#5158=CIRCLE ( 'NONE', #11095, 1.000000000000000000 ) ;
#5161=FACE_OUTER_BOUND ( 'NONE', #11995, .T. ) ;
#5165=EDGE_LOOP ( 'NONE', ( #3239, #10236, #1113, #2102 ) ) ;
#5181=AXIS2_PLACEMENT_3D ( 'NONE', #8405, #4354, #2019 ) ;
#5182=CARTESIAN_POINT ( 'NONE',  ( 0.000000000000000000, 3.000000000000000000, 5.000000000000000000 ) ) ;
#5183=VECTOR ( 'NONE', #977, 1000.000000000000227 ) ;
#5196=DIRECTION ( 'NONE',  ( 0.000000000000000000, 0.000000000000000000, -1.000000000000000000 ) ) ;
#5214=CARTESIAN_POINT ( 'NONE',  ( 53.78299299645824050, 0.000000000000000000, -4.528231303176834643 ) ) ;
#5223=CARTESIAN_POINT ( 'NONE',  ( 23.99887587215152251, 3.000000000000000000, 5.000000000000000888 ) ) ;
#5240=EDGE_CURVE ( 'NONE', #7348, #1088, #6095, .T. ) ;
#5269=DIRECTION ( 'NONE',  ( -0.000000000000000000, -1.000000000000000000, -0.000000000000000000 ) ) ;
#5276=LINE ( 'NONE', #2052, #9544 ) ;
#5281=PLANE ( 'NONE',  #2882 ) ;
#5298=CIRCLE ( 'NONE', #3971, 0.9999999999999991118 ) ;
#5317=CARTESIAN_POINT ( 'NONE',  ( 51.83140210808490167, 0.000000000000000000, -12.77460472465662988 ) ) ;
#5339=CARTESIAN_POINT ( 'NONE',  ( 41.67875868938293138, 3.000000000000000000, -6.066649533482935119 ) ) ;
#5343=ORIENTED_EDGE ( 'NONE', *, *, #7094, .T. ) ;
#5344=ADVANCED_FACE ( 'NONE', ( #925 ), #7506, .F. ) ;
#5352=DIRECTION ( 'NONE',  ( 0.000000000000000000, 0.000000000000000000, 1.000000000000000000 ) ) ;
#5363=ORIENTED_EDGE ( 'NONE', *, *, #860, .F. ) ;
#5396=EDGE_LOOP ( 'NONE', ( #1996, #359, #9297, #1867 ) ) ;
#5403=ADVANCED_FACE ( 'NONE', ( #6913 ), #5668, .F. ) ;
#5412=CARTESIAN_POINT ( 'NONE',  ( 45.60964950616533287, 3.000000000000000000, -14.50984893380129392 ) ) ;
#5414=ORIENTED_EDGE ( 'NONE', *, *, #1788, .F. ) ;
#5437=VERTEX_POINT ( 'NONE', #10079 ) ;
#5452=DIRECTION ( 'NONE',  ( 1.000000000000000000, 0.000000000000000000, 0.000000000000000000 ) ) ;
#5467=ORIENTED_EDGE ( 'NONE', *, *, #1733, .F. ) ;
#5477=DIRECTION ( 'NONE',  ( 0.000000000000000000, 0.000000000000000000, -1.000000000000000000 ) ) ;
#5489=VECTOR ( 'NONE', #11182, 1000.000000000000000 ) ;
#5513=EDGE_CURVE ( 'NONE', #464, #641, #587, .T. ) ;
#5536=EDGE_CURVE ( 'NONE', #5689, #3986, #9014, .T. ) ;
#5566=VECTOR ( 'NONE', #4521, 1000.000000000000227 ) ;
#5568=PRODUCT ( 'gripper', 'gripper', '', ( #2336 ) ) ;
#5579=ORIENTED_EDGE ( 'NONE', *, *, #12489, .T. ) ;
#5583=CIRCLE ( 'NONE', #13070, 5.000000000000000000 ) ;
#5597=ORIENTED_EDGE ( 'NONE', *, *, #12187, .F. ) ;
#5616=CARTESIAN_POINT ( 'NONE',  ( 41.29994854050690378, 3.000000000000000000, -6.141175130212632283 ) ) ;
#5619=FACE_OUTER_BOUND ( 'NONE', #7273, .T. ) ;
#5627=EDGE_LOOP ( 'NONE', ( #9216, #9100, #9438, #9271 ) ) ;
#5652=CARTESIAN_POINT ( 'NONE',  ( 54.70014691233865989, 3.000000000000000000, -3.785783530882224746 ) ) ;
#5668=PLANE ( 'NONE',  #7277 ) ;
#5681=CARTESIAN_POINT ( 'NONE',  ( 29.39270799701850123, 3.000000000000000000, -0.3930766723116408401 ) ) ;
#5689=VERTEX_POINT ( 'NONE', #8410 ) ;
#5700=DIRECTION ( 'NONE',  ( -0.000000000000000000, -1.000000000000000000, -0.000000000000000000 ) ) ;
#5708=LINE ( 'NONE', #7516, #5766 ) ;
#5709=ORIENTED_EDGE ( 'NONE', *, *, #3844, .T. ) ;
#5712=DIRECTION ( 'NONE',  ( 1.000000000000000000, 0.000000000000000000, 0.000000000000000000 ) ) ;
#5716=DIRECTION ( 'NONE',  ( 0.3802634127332040759, 0.000000000000000000, 0.9248782281665499649 ) ) ;
#5717=CARTESIAN_POINT ( 'NONE',  ( 51.38094353598858532, 0.000000000000000000, -3.436371243710653722 ) ) ;
#5719=EDGE_LOOP ( 'NONE', ( #1962, #12911, #3222, #10099 ) ) ;
#5744=EDGE_LOOP ( 'NONE', ( #7347, #3102, #6760, #3333, #4460, #3055, #372, #6429, #10098, #4187, #9785, #12952, #11869, #13203, #2299, #292, #1264, #3903, #11158, #13156, #6790, #13358, #5709, #9887, #10508, #2700, #9441 ) ) ;
#5748=ORIENTED_EDGE ( 'NONE', *, *, #1521, .F. ) ;
#5750=DIRECTION ( 'NONE',  ( -0.000000000000000000, -1.000000000000000000, -0.000000000000000000 ) ) ;
#5753=PLANE ( 'NONE',  #8791 ) ;
#5758=EDGE_CURVE ( 'NONE', #1419, #1362, #12270, .T. ) ;
#5765=ORIENTED_EDGE ( 'NONE', *, *, #13406, .F. ) ;
#5766=VECTOR ( 'NONE', #289, 1000.000000000000227 ) ;
#5777=VERTEX_POINT ( 'NONE', #9151 ) ;
#5797=ORIENTED_EDGE ( 'NONE', *, *, #6702, .F. ) ;
#5857=LINE ( 'NONE', #12280, #2913 ) ;
#5864=( LENGTH_UNIT ( ) NAMED_UNIT ( * ) SI_UNIT ( .MILLI., .METRE. ) );
#5865=DIRECTION ( 'NONE',  ( -0.6291930273682727615, 0.000000000000000000, 0.7772490812546181127 ) ) ;
#5887=VERTEX_POINT ( 'NONE', #7089 ) ;
#5892=DIRECTION ( 'NONE',  ( 1.000000000000000000, 0.000000000000000000, -0.000000000000000000 ) ) ;
#5898=VERTEX_POINT ( 'NONE', #6954 ) ;
#5919=DIRECTION ( 'NONE',  ( 0.6291930273682743158, 0.000000000000000000, -0.7772490812546168915 ) ) ;
#5923=ORIENTED_EDGE ( 'NONE', *, *, #4595, .F. ) ;
#5930=LINE ( 'NONE', #5717, #8166 ) ;
#5935=ORIENTED_EDGE ( 'NONE', *, *, #860, .T. ) ;
#5962=LINE ( 'NONE', #3680, #7113 ) ;
#5966=CARTESIAN_POINT ( 'NONE',  ( 52.34174591811297717, 3.000000000000000000, -12.24483450274845531 ) ) ;
#5967=CARTESIAN_POINT ( 'NONE',  ( 53.78299299645824050, 3.000000000000000000, -4.528231303176834643 ) ) ;
#5972=FACE_OUTER_BOUND ( 'NONE', #11296, .T. ) ;
#5979=FACE_OUTER_BOUND ( 'NONE', #2533, .T. ) ;
#5997=DIRECTION ( 'NONE',  ( -0.000000000000000000, -1.000000000000000000, -0.000000000000000000 ) ) ;
#5998=SURFACE_STYLE_USAGE ( .BOTH. , #1877 ) ;
#6000=ADVANCED_FACE ( 'NONE', ( #10389 ), #9362, .F. ) ;
#6002=AXIS2_PLACEMENT_3D ( 'NONE', #6277, #10342, #2085 ) ;
#6018=CARTESIAN_POINT ( 'NONE',  ( 49.72134184781355515, 3.000000000000000000, -3.261665100124877981 ) ) ;
#6038=AXIS2_PLACEMENT_3D ( 'NONE', #10310, #814, #7152 ) ;
#6044=DIRECTION ( 'NONE',  ( -0.9248782281665488547, -0.000000000000000000, 0.3802634127332066294 ) ) ;
#6061=LINE ( 'NONE', #7092, #2035 ) ;
#6095=LINE ( 'NONE', #10230, #13206 ) ;
#6116=CARTESIAN_POINT ( 'NONE',  ( 50.46378962010818015, 3.000000000000000000, -4.178819016005276943 ) ) ;
#6143=LINE ( 'NONE', #9176, #8452 ) ;
#6164=CARTESIAN_POINT ( 'NONE',  ( 6.123233995736766282E-16, 3.000000000000000000, -5.000000000000000000 ) ) ;
#6170=CARTESIAN_POINT ( 'NONE',  ( 45.60964950616533287, 3.000000000000000000, -14.50984893380129392 ) ) ;
#6179=VERTEX_POINT ( 'NONE', #1564 ) ;
#6188=AXIS2_PLACEMENT_3D ( 'NONE', #53, #4233, #9547 ) ;
#6193=DIRECTION ( 'NONE',  ( 0.6291930273683260522, 0.000000000000000000, -0.7772490812545749250 ) ) ;
#6216=VECTOR ( 'NONE', #8142, 1000.000000000000000 ) ;
#6237=AXIS2_PLACEMENT_3D ( 'NONE', #10429, #3050, #5196 ) ;
#6238=VECTOR ( 'NONE', #4800, 1000.000000000000000 ) ;
#6246=DIRECTION ( 'NONE',  ( 0.5610724890695777400, 0.000000000000000000, -0.8277666712360848278 ) ) ;
#6248=ADVANCED_FACE ( 'NONE', ( #4860 ), #5753, .F. ) ;
#6252=DIRECTION ( 'NONE',  ( 0.000000000000000000, 0.000000000000000000, -1.000000000000000000 ) ) ;
#6271=CARTESIAN_POINT ( 'NONE',  ( 50.46378962010818015, 3.000000000000000000, -4.178819016005276943 ) ) ;
#6274=FACE_OUTER_BOUND ( 'NONE', #10583, .T. ) ;
#6277=CARTESIAN_POINT ( 'NONE',  ( 41.29994854050690378, 0.000000000000000000, -5.141175130212632283 ) ) ;
#6289=DIRECTION ( 'NONE',  ( 0.000000000000000000, 0.000000000000000000, 1.000000000000000000 ) ) ;
#6295=ORIENTED_EDGE ( 'NONE', *, *, #8357, .F. ) ;
#6299=DIRECTION ( 'NONE',  ( 0.000000000000000000, 0.000000000000000000, 1.000000000000000000 ) ) ;
#6324=ADVANCED_FACE ( 'NONE', ( #4234 ), #2171, .F. ) ;
#6341=DIRECTION ( 'NONE',  ( 0.6291930273683203900, 0.000000000000000000, -0.7772490812545796990 ) ) ;
#6387=ORIENTED_EDGE ( 'NONE', *, *, #7418, .F. ) ;
#6389=DIRECTION ( 'NONE',  ( -0.3802634127332040759, -0.000000000000000000, -0.9248782281665499649 ) ) ;
#6391=EDGE_CURVE ( 'NONE', #11587, #5777, #4106, .T. ) ;
#6392=ADVANCED_FACE ( 'NONE', ( #13550 ), #1918, .T. ) ;
#6413=ADVANCED_FACE ( 'NONE', ( #11614 ), #13479, .F. ) ;
#6416=DIRECTION ( 'NONE',  ( 0.7772490812545874705, 0.000000000000000000, 0.6291930273683107311 ) ) ;
#6423=VECTOR ( 'NONE', #1074, 1000.000000000000000 ) ;
#6429=ORIENTED_EDGE ( 'NONE', *, *, #4172, .T. ) ;
#6434=CIRCLE ( 'NONE', #11717, 1.000000000000000888 ) ;
#6439=CARTESIAN_POINT ( 'NONE',  ( 1.836970198721030181E-16, 3.000000000000000000, 1.500000000000000222 ) ) ;
#6447=ORIENTED_EDGE ( 'NONE', *, *, #1041, .T. ) ;
#6486=LINE ( 'NONE', #1250, #12169 ) ;
#6487=ORIENTED_EDGE ( 'NONE', *, *, #7078, .T. ) ;
#6495=AXIS2_PLACEMENT_3D ( 'NONE', #13566, #2061, #11897 ) ;
#6504=ORIENTED_EDGE ( 'NONE', *, *, #1773, .F. ) ;
#6514=EDGE_CURVE ( 'NONE', #13346, #9675, #10773, .T. ) ;
#6559=CARTESIAN_POINT ( 'NONE',  ( 51.38094353598858532, 0.000000000000000000, -3.436371243710653722 ) ) ;
#6563=CARTESIAN_POINT ( 'NONE',  ( 29.02231267299996986, 3.000000000000000000, -1.321950885510182250 ) ) ;
#6589=DIRECTION ( 'NONE',  ( -0.000000000000000000, -1.000000000000000000, -0.000000000000000000 ) ) ;
#6593=ORIENTED_EDGE ( 'NONE', *, *, #9312, .F. ) ;
#6600=EDGE_CURVE ( 'NONE', #8692, #12875, #8972, .T. ) ;
#6629=DIRECTION ( 'NONE',  ( 0.000000000000000000, 1.000000000000000000, -0.000000000000000000 ) ) ;
#6650=VERTEX_POINT ( 'NONE', #7944 ) ;
#6655=AXIS2_PLACEMENT_3D ( 'NONE', #532, #6784, #2524 ) ;
#6657=CARTESIAN_POINT ( 'NONE',  ( 49.72134184781355515, 3.000000000000000000, -3.261665100124877981 ) ) ;
#6676=FACE_BOUND ( 'NONE', #3101, .T. ) ;
#6690=AXIS2_PLACEMENT_3D ( 'NONE', #1636, #2792, #1840 ) ;
#6699=ORIENTED_EDGE ( 'NONE', *, *, #1401, .F. ) ;
#6702=EDGE_CURVE ( 'NONE', #5887, #12205, #2880, .T. ) ;
#6707=COLOUR_RGB ( '',0.7803921568627451011, 0.7607843137254901578, 0.7411764705882353255 ) ;
#6711=FACE_OUTER_BOUND ( 'NONE', #12577, .T. ) ;
#6718=VERTEX_POINT ( 'NONE', #4990 ) ;
#6732=ORIENTED_EDGE ( 'NONE', *, *, #1342, .F. ) ;
#6748=VERTEX_POINT ( 'NONE', #11398 ) ;
#6749=ORIENTED_EDGE ( 'NONE', *, *, #10044, .F. ) ;
#6754=CARTESIAN_POINT ( 'NONE',  ( 0.000000000000000000, 0.000000000000000000, 0.000000000000000000 ) ) ;
#6760=ORIENTED_EDGE ( 'NONE', *, *, #9429, .T. ) ;
#6784=DIRECTION ( 'NONE',  ( -0.000000000000000000, -1.000000000000000000, -0.000000000000000000 ) ) ;
#6787=CARTESIAN_POINT ( 'NONE',  ( 50.46378962010818015, 0.000000000000000000, -4.178819016005276943 ) ) ;
#6790=ORIENTED_EDGE ( 'NONE', *, *, #9935, .T. ) ;
#6791=EDGE_LOOP ( 'NONE', ( #5765, #9062 ) ) ;
#6794=EDGE_CURVE ( 'NONE', #11616, #6718, #4093, .T. ) ;
#6806=VECTOR ( 'NONE', #11411, 1000.000000000000000 ) ;
#6835=DIRECTION ( 'NONE',  ( 0.000000000000000000, 0.000000000000000000, -1.000000000000000000 ) ) ;
#6838=EDGE_CURVE ( 'NONE', #9675, #5777, #3991, .T. ) ;
#6851=AXIS2_PLACEMENT_3D ( 'NONE', #8899, #13044, #6835 ) ;
#6855=DIRECTION ( 'NONE',  ( -0.000000000000000000, -1.000000000000000000, 0.000000000000000000 ) ) ;
#6882=VECTOR ( 'NONE', #2169, 1000.000000000000227 ) ;
#6883=AXIS2_PLACEMENT_3D ( 'NONE', #10277, #6341, #7119 ) ;
#6903=VERTEX_POINT ( 'NONE', #9721 ) ;
#6910=CARTESIAN_POINT ( 'NONE',  ( 53.78299299645824050, 3.000000000000000000, -4.528231303176834643 ) ) ;
#6913=FACE_OUTER_BOUND ( 'NONE', #7106, .T. ) ;
#6914=CIRCLE ( 'NONE', #6690, 1.000000000000000888 ) ;
#6931=DIRECTION ( 'NONE',  ( 0.000000000000000000, 0.000000000000000000, -1.000000000000000000 ) ) ;
#6935=CARTESIAN_POINT ( 'NONE',  ( 51.38094353598858532, 3.000000000000000000, -3.436371243710653722 ) ) ;
#6937=STYLED_ITEM ( 'NONE', ( #10202 ), #13452 ) ;
#6953=DIRECTION ( 'NONE',  ( -0.6291930273683253860, 0.000000000000000000, 0.7772490812545754801 ) ) ;
#6954=CARTESIAN_POINT ( 'NONE',  ( 28.56494132578241008, 3.000000000000000000, -0.9541491613812155270 ) ) ;
#6963=ORIENTED_EDGE ( 'NONE', *, *, #1901, .F. ) ;
#7014=EDGE_CURVE ( 'NONE', #10663, #8766, #5930, .T. ) ;
#7030=EDGE_CURVE ( 'NONE', #2099, #12066, #2622, .T. ) ;
#7031=EDGE_LOOP ( 'NONE', ( #12694, #2395, #6749, #9601 ) ) ;
#7035=DIRECTION ( 'NONE',  ( -0.6291930273683260522, 0.000000000000000000, 0.7772490812545750360 ) ) ;
#7050=VECTOR ( 'NONE', #10011, 1000.000000000000227 ) ;
#7060=CARTESIAN_POINT ( 'NONE',  ( 53.78299299645824050, 0.000000000000000000, -4.528231303176834643 ) ) ;
#7075=DIRECTION ( 'NONE',  ( -0.3802634127332040759, -0.000000000000000000, -0.9248782281665499649 ) ) ;
#7077=FACE_OUTER_BOUND ( 'NONE', #2759, .T. ) ;
#7078=EDGE_CURVE ( 'NONE', #578, #6748, #9436, .T. ) ;
#7088=CARTESIAN_POINT ( 'NONE',  ( 49.72134184781355515, 3.000000000000000000, -3.261665100124877981 ) ) ;
#7089=CARTESIAN_POINT ( 'NONE',  ( 22.00000000000000000, 0.000000000000000000, -1.500000000000000666 ) ) ;
#7092=CARTESIAN_POINT ( 'NONE',  ( 46.02418392430381999, 3.000000000000000000, -15.41988256844266836 ) ) ;
#7094=EDGE_CURVE ( 'NONE', #6748, #13415, #7307, .T. ) ;
#7097=ORIENTED_EDGE ( 'NONE', *, *, #596, .F. ) ;
#7106=EDGE_LOOP ( 'NONE', ( #10746, #6963, #9705, #7748 ) ) ;
#7108=LINE ( 'NONE', #3786, #9857 ) ;
#7113=VECTOR ( 'NONE', #6044, 1000.000000000000227 ) ;
#7119=DIRECTION ( 'NONE',  ( -0.7772490812545796990, 0.000000000000000000, -0.6291930273683203900 ) ) ;
#7124=VECTOR ( 'NONE', #11131, 1000.000000000000000 ) ;
#7131=DIRECTION ( 'NONE',  ( -0.000000000000000000, -1.000000000000000000, -0.000000000000000000 ) ) ;
#7135=DIRECTION ( 'NONE',  ( 0.7772490812545826966, 0.000000000000000000, 0.6291930273683166153 ) ) ;
#7152=DIRECTION ( 'NONE',  ( 0.9100336346413741007, 0.000000000000000000, 0.4145344181384821858 ) ) ;
#7171=ORIENTED_EDGE ( 'NONE', *, *, #12605, .T. ) ;
#7175=VERTEX_POINT ( 'NONE', #7243 ) ;
#7188=CARTESIAN_POINT ( 'NONE',  ( 52.34174591811297717, 3.000000000000000000, -12.24483450274845531 ) ) ;
#7196=LINE ( 'NONE', #11598, #6216 ) ;
#7210=EDGE_CURVE ( 'NONE', #12572, #5437, #7950, .T. ) ;
#7217=DIRECTION ( 'NONE',  ( -0.8277666712360849388, 0.000000000000000000, -0.5610724890695777400 ) ) ;
#7220=DIRECTION ( 'NONE',  ( 0.000000000000000000, 0.000000000000000000, 1.000000000000000000 ) ) ;
#7231=APPLICATION_CONTEXT ( 'automotive_design' ) ;
#7243=CARTESIAN_POINT ( 'NONE',  ( 52.34174591811297717, 0.000000000000000000, -12.24483450274845531 ) ) ;
#7254=DIRECTION ( 'NONE',  ( 0.7772490812545771455, 0.000000000000000000, 0.6291930273683233876 ) ) ;
#7267=ORIENTED_EDGE ( 'NONE', *, *, #4144, .F. ) ;
#7268=VERTEX_POINT ( 'NONE', #3293 ) ;
#7273=EDGE_LOOP ( 'NONE', ( #13519, #8442, #6387, #1683 ) ) ;
#7277=AXIS2_PLACEMENT_3D ( 'NONE', #10146, #7938, #3734 ) ;
#7280=VECTOR ( 'NONE', #11599, 1000.000000000000000 ) ;
#7307=LINE ( 'NONE', #8198, #4214 ) ;
#7344=DIRECTION ( 'NONE',  ( -0.000000000000000000, -1.000000000000000000, -0.000000000000000000 ) ) ;
#7347=ORIENTED_EDGE ( 'NONE', *, *, #7418, .T. ) ;
#7348=VERTEX_POINT ( 'NONE', #8666 ) ;
#7355=EDGE_CURVE ( 'NONE', #13143, #6903, #9503, .T. ) ;
#7357=SHAPE_DEFINITION_REPRESENTATION ( #7775, #8539 ) ;
#7379=LINE ( 'NONE', #9636, #3963 ) ;
#7383=ORIENTED_EDGE ( 'NONE', *, *, #5513, .F. ) ;
#7390=ORIENTED_EDGE ( 'NONE', *, *, #5005, .T. ) ;
#7407=ORIENTED_EDGE ( 'NONE', *, *, #9849, .F. ) ;
#7418=EDGE_CURVE ( 'NONE', #5898, #8692, #7743, .T. ) ;
#7431=ORIENTED_EDGE ( 'NONE', *, *, #9312, .T. ) ;
#7434=CARTESIAN_POINT ( 'NONE',  ( 19.65244806805498001, 3.000000000000000000, -5.000000000000000000 ) ) ;
#7479=CYLINDRICAL_SURFACE ( 'NONE', #66, 1.000000000000000888 ) ;
#7481=LINE ( 'NONE', #11686, #5566 ) ;
#7495=ORIENTED_EDGE ( 'NONE', *, *, #10386, .T. ) ;
#7504=EDGE_CURVE ( 'NONE', #3318, #10776, #12413, .T. ) ;
#7506=CYLINDRICAL_SURFACE ( 'NONE', #7696, 1.500000000000000666 ) ;
#7510=EDGE_CURVE ( 'NONE', #10535, #7268, #826, .T. ) ;
#7516=CARTESIAN_POINT ( 'NONE',  ( 47.14458624375820506, 3.000000000000000000, -3.829406728833672613 ) ) ;
#7517=VECTOR ( 'NONE', #7135, 1000.000000000000227 ) ;
#7522=EDGE_CURVE ( 'NONE', #12066, #11648, #6061, .T. ) ;
#7526=AXIS2_PLACEMENT_3D ( 'NONE', #1511, #3772, #1724 ) ;
#7556=AXIS2_PLACEMENT_3D ( 'NONE', #2865, #7217, #9060 ) ;
#7570=ORIENTED_EDGE ( 'NONE', *, *, #7522, .F. ) ;
#7572=AXIS2_PLACEMENT_3D ( 'NONE', #5681, #5750, #2649 ) ;
#7577=CARTESIAN_POINT ( 'NONE',  ( 22.00000000000000000, 3.000000000000000000, 0.000000000000000000 ) ) ;
#7583=ORIENTED_EDGE ( 'NONE', *, *, #2892, .F. ) ;
#7584=( GEOMETRIC_REPRESENTATION_CONTEXT ( 3 ) GLOBAL_UNCERTAINTY_ASSIGNED_CONTEXT ( ( #3777 ) ) GLOBAL_UNIT_ASSIGNED_CONTEXT ( ( #12389, #9340, #9133 ) ) REPRESENTATION_CONTEXT ( 'NONE', 'WORKASPACE' ) );
#7618=ORIENTED_EDGE ( 'NONE', *, *, #12533, .F. ) ;
#7630=LINE ( 'NONE', #4387, #13330 ) ;
#7643=DIRECTION ( 'NONE',  ( 0.000000000000000000, 0.000000000000000000, 1.000000000000000000 ) ) ;
#7650=CARTESIAN_POINT ( 'NONE',  ( 45.22938609343211880, 3.000000000000000000, -15.43472716196784233 ) ) ;
#7655=CARTESIAN_POINT ( 'NONE',  ( 41.29994854050690378, 3.000000000000000000, -5.141175130212632283 ) ) ;
#7662=PLANE ( 'NONE',  #12172 ) ;
#7683=DIRECTION ( 'NONE',  ( 0.000000000000000000, 0.000000000000000000, 1.000000000000000000 ) ) ;
#7696=AXIS2_PLACEMENT_3D ( 'NONE', #7577, #5120, #11779 ) ;
#7716=EDGE_LOOP ( 'NONE', ( #13247, #9383, #9856, #7764 ) ) ;
#7724=PLANE ( 'NONE',  #1210 ) ;
#7742=VECTOR ( 'NONE', #5072, 1000.000000000000000 ) ;
#7743=CIRCLE ( 'NONE', #7526, 1.000000000000000888 ) ;
#7748=ORIENTED_EDGE ( 'NONE', *, *, #1445, .T. ) ;
#7754=CIRCLE ( 'NONE', #6655, 1.000000000000000888 ) ;
#7762=VERTEX_POINT ( 'NONE', #7060 ) ;
#7764=ORIENTED_EDGE ( 'NONE', *, *, #2780, .T. ) ;
#7775=PRODUCT_DEFINITION_SHAPE ( 'NONE', 'NONE',  #1605 ) ;
#7781=VERTEX_POINT ( 'NONE', #593 ) ;
#7799=EDGE_LOOP ( 'NONE', ( #610, #1265, #7407, #3053 ) ) ;
#7822=CARTESIAN_POINT ( 'NONE',  ( 52.12339130828321032, 3.000000000000000000, -4.353525159591052685 ) ) ;
#7869=CARTESIAN_POINT ( 'NONE',  ( 0.000000000000000000, 3.000000000000000000, 0.000000000000000000 ) ) ;
#7899=DIRECTION ( 'NONE',  ( 0.000000000000000000, 0.000000000000000000, -1.000000000000000000 ) ) ;
#7917=DIRECTION ( 'NONE',  ( -0.000000000000000000, -1.000000000000000000, -0.000000000000000000 ) ) ;
#7928=ORIENTED_EDGE ( 'NONE', *, *, #12521, .T. ) ;
#7933=CARTESIAN_POINT ( 'NONE',  ( 41.29994854050690378, 0.000000000000000000, -6.141175130212632283 ) ) ;
#7938=DIRECTION ( 'NONE',  ( 0.6291930273683166153, 0.000000000000000000, -0.7772490812545826966 ) ) ;
#7944=CARTESIAN_POINT ( 'NONE',  ( 28.56494132578241008, 0.000000000000000000, -0.9541491613812155270 ) ) ;
#7950=CIRCLE ( 'NONE', #2026, 1.000000000000000888 ) ;
#7961=CARTESIAN_POINT ( 'NONE',  ( 0.000000000000000000, 3.000000000000000000, -1.500000000000000222 ) ) ;
#8022=ORIENTED_EDGE ( 'NONE', *, *, #8357, .T. ) ;
#8084=DIRECTION ( 'NONE',  ( 0.000000000000000000, 1.000000000000000000, 0.000000000000000000 ) ) ;
#8097=ADVANCED_FACE ( 'NONE', ( #3453 ), #7662, .F. ) ;
#8098=CYLINDRICAL_SURFACE ( 'NONE', #11727, 1.000000000000000888 ) ;
#8102=EDGE_CURVE ( 'NONE', #12066, #11098, #6434, .T. ) ;
#8103=FACE_OUTER_BOUND ( 'NONE', #4424, .T. ) ;
#8123=AXIS2_PLACEMENT_3D ( 'NONE', #8659, #4603, #10877 ) ;
#8137=EDGE_LOOP ( 'NONE', ( #13222, #4023, #2144, #830 ) ) ;
#8138=DIRECTION ( 'NONE',  ( 0.6291930273682727615, 0.000000000000000000, -0.7772490812546181127 ) ) ;
#8142=DIRECTION ( 'NONE',  ( -0.9100336346413742117, -0.000000000000000000, -0.4145344181384821858 ) ) ;
#8155=ORIENTED_EDGE ( 'NONE', *, *, #8848, .F. ) ;
#8166=VECTOR ( 'NONE', #12074, 1000.000000000000000 ) ;
#8186=VECTOR ( 'NONE', #8138, 1000.000000000000000 ) ;
#8198=CARTESIAN_POINT ( 'NONE',  ( 20.03271148078819408, 0.000000000000000000, -5.075121771833452478 ) ) ;
#8202=ADVANCED_FACE ( 'NONE', ( #3656, #1606, #2694 ), #3592, .T. ) ;
#8209=AXIS2_PLACEMENT_3D ( 'NONE', #8700, #12854, #9735 ) ;
#8214=LINE ( 'NONE', #9393, #11658 ) ;
#8216=CYLINDRICAL_SURFACE ( 'NONE', #6237, 1.500000000000000222 ) ;
#8234=DIRECTION ( 'NONE',  ( -0.000000000000000000, -1.000000000000000000, -0.000000000000000000 ) ) ;
#8237=AXIS2_PLACEMENT_3D ( 'NONE', #1411, #584, #4779 ) ;
#8243=LINE ( 'NONE', #5214, #10848 ) ;
#8260=VERTEX_POINT ( 'NONE', #498 ) ;
#8267=PRODUCT_DEFINITION_FORMATION_WITH_SPECIFIED_SOURCE ( 'ANY', '', #5568, .NOT_KNOWN. ) ;
#8284=FACE_OUTER_BOUND ( 'NONE', #1628, .T. ) ;
#8298=EDGE_CURVE ( 'NONE', #1592, #8260, #12501, .T. ) ;
#8302=CARTESIAN_POINT ( 'NONE',  ( 40.92955321648837241, 3.000000000000000000, -6.070049343411170639 ) ) ;
#8311=CARTESIAN_POINT ( 'NONE',  ( 0.000000000000000000, 0.000000000000000000, 0.000000000000000000 ) ) ;
#8357=EDGE_CURVE ( 'NONE', #2239, #7175, #9384, .T. ) ;
#8373=CARTESIAN_POINT ( 'NONE',  ( 41.67875868938293138, 3.000000000000000000, -6.066649533482935119 ) ) ;
#8375=CARTESIAN_POINT ( 'NONE',  ( 19.65244806805498357, 0.000000000000000000, -6.000000000000000000 ) ) ;
#8389=CARTESIAN_POINT ( 'NONE',  ( 0.000000000000000000, 0.000000000000000000, 5.000000000000000000 ) ) ;
#8392=CARTESIAN_POINT ( 'NONE',  ( 23.99887587215152607, 3.000000000000000000, 4.000000000000000000 ) ) ;
#8405=CARTESIAN_POINT ( 'NONE',  ( 22.00000000000000000, 3.000000000000000000, 0.000000000000000000 ) ) ;
#8410=CARTESIAN_POINT ( 'NONE',  ( 23.99887587215152251, 0.000000000000000000, 5.000000000000000888 ) ) ;
#8416=ADVANCED_FACE ( 'NONE', ( #6274 ), #3173, .F. ) ;
#8442=ORIENTED_EDGE ( 'NONE', *, *, #9053, .F. ) ;
#8452=VECTOR ( 'NONE', #7254, 1000.000000000000227 ) ;
#8457=LINE ( 'NONE', #10474, #3789 ) ;
#8458=ORIENTED_EDGE ( 'NONE', *, *, #10386, .F. ) ;
#8471=ORIENTED_EDGE ( 'NONE', *, *, #6514, .T. ) ;
#8476=ORIENTED_EDGE ( 'NONE', *, *, #6702, .T. ) ;
#8489=ORIENTED_EDGE ( 'NONE', *, *, #7504, .T. ) ;
#8513=FACE_OUTER_BOUND ( 'NONE', #7716, .T. ) ;
#8539=SHAPE_REPRESENTATION ( 'gripper', ( #10007 ), #12883 ) ;
#8543=CARTESIAN_POINT ( 'NONE',  ( 0.000000000000000000, 3.000000000000000000, -5.000000000000000000 ) ) ;
#8579=AXIS2_PLACEMENT_3D ( 'NONE', #13563, #2058, #6252 ) ;
#8584=CARTESIAN_POINT ( 'NONE',  ( 6.123233995736766282E-16, 0.000000000000000000, -5.000000000000000000 ) ) ;
#8590=CIRCLE ( 'NONE', #662, 1.500000000000000666 ) ;
#8610=VECTOR ( 'NONE', #5700, 1000.000000000000000 ) ;
#8622=VECTOR ( 'NONE', #6416, 1000.000000000000114 ) ;
#8652=ORIENTED_EDGE ( 'NONE', *, *, #12916, .T. ) ;
#8659=CARTESIAN_POINT ( 'NONE',  ( 29.39270799701850123, 3.000000000000000000, -0.3930766723116408401 ) ) ;
#8663=CIRCLE ( 'NONE', #11757, 1.000000000000000888 ) ;
#8665=CARTESIAN_POINT ( 'NONE',  ( 45.60964950616533287, 3.000000000000000000, -15.50984893380129392 ) ) ;
#8666=CARTESIAN_POINT ( 'NONE',  ( 19.65244806805498001, 0.000000000000000000, -5.000000000000000000 ) ) ;
#8689=FACE_OUTER_BOUND ( 'NONE', #12129, .T. ) ;
#8692=VERTEX_POINT ( 'NONE', #4057 ) ;
#8700=CARTESIAN_POINT ( 'NONE',  ( 48.06174015963858892, 3.000000000000000000, -3.086958956539055166 ) ) ;
#8741=ORIENTED_EDGE ( 'NONE', *, *, #6838, .T. ) ;
#8763=AXIS2_PLACEMENT_3D ( 'NONE', #2826, #9090, #13309 ) ;
#8766=VERTEX_POINT ( 'NONE', #9568 ) ;
#8791=AXIS2_PLACEMENT_3D ( 'NONE', #534, #12256, #664 ) ;
#8830=ORIENTED_EDGE ( 'NONE', *, *, #2278, .F. ) ;
#8842=AXIS2_PLACEMENT_3D ( 'NONE', #12586, #12526, #6299 ) ;
#8848=EDGE_CURVE ( 'NONE', #2099, #10532, #2187, .T. ) ;
#8899=CARTESIAN_POINT ( 'NONE',  ( 41.29994854050690378, 0.000000000000000000, -5.141175130212632283 ) ) ;
#8900=VECTOR ( 'NONE', #1863, 1000.000000000000000 ) ;
#8902=FACE_OUTER_BOUND ( 'NONE', #5165, .T. ) ;
#8914=LINE ( 'NONE', #11059, #7124 ) ;
#8953=DIRECTION ( 'NONE',  ( -0.9248782281665499649, 0.000000000000000000, 0.3802634127332040759 ) ) ;
#8961=ADVANCED_FACE ( 'NONE', ( #7077 ), #5008, .F. ) ;
#8972=LINE ( 'NONE', #2784, #11472 ) ;
#8983=EDGE_CURVE ( 'NONE', #10283, #7762, #9202, .T. ) ;
#9000=CARTESIAN_POINT ( 'NONE',  ( 55.44259468463320673, 3.000000000000000000, -4.702937446762657459 ) ) ;
#9014=CIRCLE ( 'NONE', #4403, 1.000000000000000888 ) ;
#9039=CYLINDRICAL_SURFACE ( 'NONE', #3365, 1.500000000000000222 ) ;
#9043=DIRECTION ( 'NONE',  ( -0.000000000000000000, -1.000000000000000000, -0.000000000000000000 ) ) ;
#9053=EDGE_CURVE ( 'NONE', #8692, #1419, #12259, .T. ) ;
#9060=DIRECTION ( 'NONE',  ( -0.5610724890695777400, 0.000000000000000000, 0.8277666712360849388 ) ) ;
#9062=ORIENTED_EDGE ( 'NONE', *, *, #5005, .F. ) ;
#9074=CARTESIAN_POINT ( 'NONE',  ( 48.06174015963858892, 3.000000000000000000, -3.086958956539055166 ) ) ;
#9090=DIRECTION ( 'NONE',  ( 0.000000000000000000, 1.000000000000000000, -0.000000000000000000 ) ) ;
#9100=ORIENTED_EDGE ( 'NONE', *, *, #12605, .F. ) ;
#9111=ADVANCED_FACE ( 'NONE', ( #8902 ), #2575, .F. ) ;
#9118=DIRECTION ( 'NONE',  ( -0.000000000000000000, -1.000000000000000000, -0.000000000000000000 ) ) ;
#9119=VECTOR ( 'NONE', #201, 1000.000000000000000 ) ;
#9129=AXIS2_PLACEMENT_3D ( 'NONE', #11451, #9391, #2088 ) ;
#9133=( NAMED_UNIT ( * ) SI_UNIT ( $, .STERADIAN. ) SOLID_ANGLE_UNIT ( ) );
#9134=LINE ( 'NONE', #739, #6882 ) ;
#9146=VECTOR ( 'NONE', #5997, 1000.000000000000000 ) ;
#9151=CARTESIAN_POINT ( 'NONE',  ( 0.000000000000000000, 0.000000000000000000, -1.500000000000000222 ) ) ;
#9176=CARTESIAN_POINT ( 'NONE',  ( 50.46378962010818015, 0.000000000000000000, -4.178819016005276943 ) ) ;
#9202=LINE ( 'NONE', #5967, #9317 ) ;
#9216=ORIENTED_EDGE ( 'NONE', *, *, #12533, .T. ) ;
#9221=VECTOR ( 'NONE', #12194, 1000.000000000000000 ) ;
#9224=DIRECTION ( 'NONE',  ( -0.000000000000000000, -1.000000000000000000, -0.000000000000000000 ) ) ;
#9271=ORIENTED_EDGE ( 'NONE', *, *, #7510, .T. ) ;
#9297=ORIENTED_EDGE ( 'NONE', *, *, #3657, .T. ) ;
#9308=DIRECTION ( 'NONE',  ( -0.000000000000000000, -1.000000000000000000, -0.000000000000000000 ) ) ;
#9312=EDGE_CURVE ( 'NONE', #10532, #11648, #7196, .T. ) ;
#9317=VECTOR ( 'NONE', #3897, 1000.000000000000000 ) ;
#9339=CIRCLE ( 'NONE', #4053, 1.000000000000000888 ) ;
#9340=( NAMED_UNIT ( * ) PLANE_ANGLE_UNIT ( ) SI_UNIT ( $, .RADIAN. ) );
#9362=CYLINDRICAL_SURFACE ( 'NONE', #8579, 1.500000000000000666 ) ;
#9365=CYLINDRICAL_SURFACE ( 'NONE', #6495, 5.000000000000000000 ) ;
#9383=ORIENTED_EDGE ( 'NONE', *, *, #1445, .F. ) ;
#9384=LINE ( 'NONE', #7188, #5129 ) ;
#9391=DIRECTION ( 'NONE',  ( -0.000000000000000000, -1.000000000000000000, -0.000000000000000000 ) ) ;
#9393=CARTESIAN_POINT ( 'NONE',  ( 40.92955321648837241, 3.000000000000000000, -6.070049343411170639 ) ) ;
#9427=ORIENTED_EDGE ( 'NONE', *, *, #10118, .F. ) ;
#9429=EDGE_CURVE ( 'NONE', #12875, #344, #2246, .T. ) ;
#9436=LINE ( 'NONE', #15, #9496 ) ;
#9438=ORIENTED_EDGE ( 'NONE', *, *, #3473, .F. ) ;
#9441=ORIENTED_EDGE ( 'NONE', *, *, #1569, .T. ) ;
#9471=AXIS2_PLACEMENT_3D ( 'NONE', #11777, #10740, #3429 ) ;
#9476=VECTOR ( 'NONE', #7344, 1000.000000000000000 ) ;
#9487=DIRECTION ( 'NONE',  ( -0.7772490812545752581, 0.000000000000000000, -0.6291930273683257191 ) ) ;
#9496=VECTOR ( 'NONE', #1942, 1000.000000000000000 ) ;
#9503=LINE ( 'NONE', #9000, #8610 ) ;
#9512=EDGE_CURVE ( 'NONE', #10283, #291, #3447, .T. ) ;
#9540=EDGE_CURVE ( 'NONE', #11098, #12786, #488, .T. ) ;
#9544=VECTOR ( 'NONE', #6246, 1000.000000000000000 ) ;
#9547=DIRECTION ( 'NONE',  ( 0.000000000000000000, 0.000000000000000000, 1.000000000000000000 ) ) ;
#9560=DIRECTION ( 'NONE',  ( 0.000000000000000000, 1.000000000000000000, -0.000000000000000000 ) ) ;
#9568=CARTESIAN_POINT ( 'NONE',  ( 52.12339130828321032, 0.000000000000000000, -4.353525159591052685 ) ) ;
#9596=DIRECTION ( 'NONE',  ( 0.000000000000000000, 0.000000000000000000, 1.000000000000000000 ) ) ;
#9601=ORIENTED_EDGE ( 'NONE', *, *, #1901, .T. ) ;
#9607=ADVANCED_FACE ( 'NONE', ( #1738 ), #3787, .F. ) ;
#9618=ORIENTED_EDGE ( 'NONE', *, *, #388, .F. ) ;
#9625=LINE ( 'NONE', #2392, #11775 ) ;
#9636=CARTESIAN_POINT ( 'NONE',  ( 48.80418793193314997, 3.000000000000000000, -4.004112872419501201 ) ) ;
#9657=DIRECTION ( 'NONE',  ( 0.000000000000000000, 1.000000000000000000, 0.000000000000000000 ) ) ;
#9675=VERTEX_POINT ( 'NONE', #10271 ) ;
#9697=ADVANCED_FACE ( 'NONE', ( #5029 ), #11, .F. ) ;
#9705=ORIENTED_EDGE ( 'NONE', *, *, #6794, .F. ) ;
#9721=CARTESIAN_POINT ( 'NONE',  ( 55.44259468463320673, 0.000000000000000000, -4.702937446762657459 ) ) ;
#9724=CARTESIAN_POINT ( 'NONE',  ( 45.60964950616533287, 3.000000000000000000, -14.50984893380129392 ) ) ;
#9735=DIRECTION ( 'NONE',  ( -0.6291930273682743158, 0.000000000000000000, 0.7772490812546168915 ) ) ;
#9756=LINE ( 'NONE', #11692, #9119 ) ;
#9767=AXIS2_PLACEMENT_3D ( 'NONE', #11060, #7683, #5892 ) ;
#9785=ORIENTED_EDGE ( 'NONE', *, *, #4789, .T. ) ;
#9830=ORIENTED_EDGE ( 'NONE', *, *, #4743, .F. ) ;
#9844=EDGE_CURVE ( 'NONE', #8260, #5689, #11967, .T. ) ;
#9849=EDGE_CURVE ( 'NONE', #2082, #1008, #7754, .T. ) ;
#9856=ORIENTED_EDGE ( 'NONE', *, *, #4789, .F. ) ;
#9857=VECTOR ( 'NONE', #9224, 1000.000000000000000 ) ;
#9887=ORIENTED_EDGE ( 'NONE', *, *, #12721, .T. ) ;
#9904=CIRCLE ( 'NONE', #12576, 1.000000000000000888 ) ;
#9935=EDGE_CURVE ( 'NONE', #578, #2082, #5962, .T. ) ;
#9938=ADVANCED_FACE ( 'NONE', ( #1637 ), #8098, .F. ) ;
#9941=CIRCLE ( 'NONE', #6002, 1.000000000000000000 ) ;
#9959=DIRECTION ( 'NONE',  ( 0.000000000000000000, 0.000000000000000000, 1.000000000000000000 ) ) ;
#9979=ORIENTED_EDGE ( 'NONE', *, *, #11210, .F. ) ;
#9987=VERTEX_POINT ( 'NONE', #13130 ) ;
#10007=AXIS2_PLACEMENT_3D ( 'NONE', #6754, #3381, #5712 ) ;
#10011=DIRECTION ( 'NONE',  ( 0.9254744032703045020, 0.000000000000000000, 0.3788101488760216018 ) ) ;
#10034=CARTESIAN_POINT ( 'NONE',  ( 0.000000000000000000, 3.000000000000000000, 0.000000000000000000 ) ) ;
#10037=EDGE_LOOP ( 'NONE', ( #2203, #8155, #1781, #8022 ) ) ;
#10041=ORIENTED_EDGE ( 'NONE', *, *, #8298, .T. ) ;
#10044=EDGE_CURVE ( 'NONE', #6718, #10283, #9134, .T. ) ;
#10046=CARTESIAN_POINT ( 'NONE',  ( 29.02231267299996986, 0.000000000000000000, -1.321950885510182250 ) ) ;
#10062=( NAMED_UNIT ( * ) PLANE_ANGLE_UNIT ( ) SI_UNIT ( $, .RADIAN. ) );
#10079=CARTESIAN_POINT ( 'NONE',  ( 24.82664254338761722, 3.000000000000000000, 4.561072489069574409 ) ) ;
#10095=LINE ( 'NONE', #12998, #11972 ) ;
#10098=ORIENTED_EDGE ( 'NONE', *, *, #4743, .T. ) ;
#10099=ORIENTED_EDGE ( 'NONE', *, *, #3899, .T. ) ;
#10107=DIRECTION ( 'NONE',  ( -0.000000000000000000, -1.000000000000000000, 0.000000000000000000 ) ) ;
#10118=EDGE_CURVE ( 'NONE', #1088, #8260, #295, .T. ) ;
#10129=CARTESIAN_POINT ( 'NONE',  ( 48.06174015963858892, 0.000000000000000000, -3.086958956539055166 ) ) ;
#10146=CARTESIAN_POINT ( 'NONE',  ( 52.12339130828321032, 3.000000000000000000, -4.353525159591052685 ) ) ;
#10165=AXIS2_PLACEMENT_3D ( 'NONE', #5652, #1671, #5865 ) ;
#10169=ORIENTED_EDGE ( 'NONE', *, *, #2388, .F. ) ;
#10202=PRESENTATION_STYLE_ASSIGNMENT (( #5998 ) ) ;
#10230=CARTESIAN_POINT ( 'NONE',  ( 0.000000000000000000, 0.000000000000000000, -5.000000000000000000 ) ) ;
#10232=CARTESIAN_POINT ( 'NONE',  ( 52.12339130828321032, 3.000000000000000000, -4.353525159591052685 ) ) ;
#10236=ORIENTED_EDGE ( 'NONE', *, *, #3899, .F. ) ;
#10241=CARTESIAN_POINT ( 'NONE',  ( 51.83140210808490167, 3.000000000000000000, -12.77460472465662988 ) ) ;
#10243=DIRECTION ( 'NONE',  ( -0.000000000000000000, -1.000000000000000000, -0.000000000000000000 ) ) ;
#10253=ORIENTED_EDGE ( 'NONE', *, *, #2278, .T. ) ;
#10254=CARTESIAN_POINT ( 'NONE',  ( 24.82664254338761722, 3.000000000000000000, 4.561072489069574409 ) ) ;
#10271=CARTESIAN_POINT ( 'NONE',  ( 1.836970198721030181E-16, 0.000000000000000000, 1.500000000000000222 ) ) ;
#10277=CARTESIAN_POINT ( 'NONE',  ( 48.80418793193314997, 3.000000000000000000, -4.004112872419501201 ) ) ;
#10282=LINE ( 'NONE', #11177, #728 ) ;
#10283=VERTEX_POINT ( 'NONE', #11815 ) ;
#10291=CARTESIAN_POINT ( 'NONE',  ( 41.67875868938293138, 3.000000000000000000, -6.066649533482935119 ) ) ;
#10296=ADVANCED_FACE ( 'NONE', ( #6711 ), #2312, .F. ) ;
#10310=CARTESIAN_POINT ( 'NONE',  ( 46.02418392430381999, 3.000000000000000000, -15.41988256844266658 ) ) ;
#10315=ORIENTED_EDGE ( 'NONE', *, *, #9540, .T. ) ;
#10335=DIRECTION ( 'NONE',  ( -0.9248782281665488547, -0.000000000000000000, 0.3802634127332066294 ) ) ;
#10340=ORIENTED_EDGE ( 'NONE', *, *, #12489, .F. ) ;
#10342=DIRECTION ( 'NONE',  ( -0.000000000000000000, -1.000000000000000000, 0.000000000000000000 ) ) ;
#10377=ORIENTED_EDGE ( 'NONE', *, *, #666, .T. ) ;
#10380=DIRECTION ( 'NONE',  ( 0.7772490812545874705, 0.000000000000000000, 0.6291930273683107311 ) ) ;
#10386=EDGE_CURVE ( 'NONE', #641, #7781, #13119, .T. ) ;
#10389=FACE_OUTER_BOUND ( 'NONE', #10948, .T. ) ;
#10427=DIRECTION ( 'NONE',  ( 0.000000000000000000, 0.000000000000000000, 1.000000000000000000 ) ) ;
#10429=CARTESIAN_POINT ( 'NONE',  ( 0.000000000000000000, 3.000000000000000000, 0.000000000000000000 ) ) ;
#10432=ORIENTED_EDGE ( 'NONE', *, *, #12896, .F. ) ;
#10449=CARTESIAN_POINT ( 'NONE',  ( 41.67875868938293138, 3.000000000000000000, -6.066649533482935119 ) ) ;
#10451=VECTOR ( 'NONE', #5452, 1000.000000000000000 ) ;
#10455=ADVANCED_FACE ( 'NONE', ( #589 ), #9039, .F. ) ;
#10474=CARTESIAN_POINT ( 'NONE',  ( 53.04054522416362261, 0.000000000000000000, -3.611077387296437013 ) ) ;
#10494=CYLINDRICAL_SURFACE ( 'NONE', #9129, 1.000000000000000000 ) ;
#10508=ORIENTED_EDGE ( 'NONE', *, *, #11927, .T. ) ;
#10531=ORIENTED_EDGE ( 'NONE', *, *, #7210, .F. ) ;
#10532=VERTEX_POINT ( 'NONE', #5317 ) ;
#10535=VERTEX_POINT ( 'NONE', #10291 ) ;
#10575=ADVANCED_FACE ( 'NONE', ( #8284 ), #8216, .F. ) ;
#10579=DIRECTION ( 'NONE',  ( 0.3788101488760216018, 0.000000000000000000, -0.9254744032703046130 ) ) ;
#10583=EDGE_LOOP ( 'NONE', ( #7495, #13173, #4260, #4027 ) ) ;
#10593=CIRCLE ( 'NONE', #6851, 1.000000000000000000 ) ;
#10602=ORIENTED_EDGE ( 'NONE', *, *, #3217, .T. ) ;
#10618=AXIS2_PLACEMENT_3D ( 'NONE', #6910, #437, #646 ) ;
#10663=VERTEX_POINT ( 'NONE', #6559 ) ;
#10701=CARTESIAN_POINT ( 'NONE',  ( 0.000000000000000000, 0.000000000000000000, 0.000000000000000000 ) ) ;
#10724=LINE ( 'NONE', #2385, #1850 ) ;
#10730=CARTESIAN_POINT ( 'NONE',  ( 23.99887587215152251, 3.000000000000000000, 5.000000000000000888 ) ) ;
#10740=DIRECTION ( 'NONE',  ( 0.000000000000000000, 1.000000000000000000, -0.000000000000000000 ) ) ;
#10745=DIRECTION ( 'NONE',  ( 0.000000000000000000, 0.000000000000000000, -1.000000000000000000 ) ) ;
#10746=ORIENTED_EDGE ( 'NONE', *, *, #1733, .T. ) ;
#10762=DIRECTION ( 'NONE',  ( -0.3703953240185315909, 0.000000000000000000, -0.9288742131985401329 ) ) ;
#10773=LINE ( 'NONE', #6439, #11248 ) ;
#10776=VERTEX_POINT ( 'NONE', #10129 ) ;
#10781=CARTESIAN_POINT ( 'NONE',  ( 24.82664254338761722, 0.000000000000000000, 4.561072489069574409 ) ) ;
#10802=AXIS2_PLACEMENT_3D ( 'NONE', #515, #4717, #6289 ) ;
#10815=ADVANCED_FACE ( 'NONE', ( #702 ), #12073, .F. ) ;
#10832=DIRECTION ( 'NONE',  ( 0.000000000000000000, 0.000000000000000000, -1.000000000000000000 ) ) ;
#10842=CARTESIAN_POINT ( 'NONE',  ( 52.34174591811297717, 3.000000000000000000, -12.24483450274845531 ) ) ;
#10848=VECTOR ( 'NONE', #10380, 1000.000000000000114 ) ;
#10877=DIRECTION ( 'NONE',  ( 0.000000000000000000, -0.000000000000000000, -1.000000000000000000 ) ) ;
#10885=DIRECTION ( 'NONE',  ( -0.000000000000000000, -1.000000000000000000, -0.000000000000000000 ) ) ;
#10920=ORIENTED_EDGE ( 'NONE', *, *, #4568, .T. ) ;
#10921=ORIENTED_EDGE ( 'NONE', *, *, #7030, .F. ) ;
#10923=FACE_OUTER_BOUND ( 'NONE', #4080, .T. ) ;
#10948=EDGE_LOOP ( 'NONE', ( #11802, #1075, #5797, #7583 ) ) ;
#10973=CARTESIAN_POINT ( 'NONE',  ( 1.836970198721030181E-16, 3.000000000000000000, 1.500000000000000222 ) ) ;
#10999=DIRECTION ( 'NONE',  ( 0.000000000000000000, 0.000000000000000000, -1.000000000000000000 ) ) ;
#11005=FACE_BOUND ( 'NONE', #6791, .T. ) ;
#11054=ORIENTED_EDGE ( 'NONE', *, *, #5240, .F. ) ;
#11059=CARTESIAN_POINT ( 'NONE',  ( 53.04054522416362261, 3.000000000000000000, -3.611077387296437013 ) ) ;
#11060=CARTESIAN_POINT ( 'NONE',  ( 0.000000000000000000, 3.000000000000000000, -5.000000000000000000 ) ) ;
#11095=AXIS2_PLACEMENT_3D ( 'NONE', #3679, #6855, #6931 ) ;
#11098=VERTEX_POINT ( 'NONE', #8665 ) ;
#11124=DIRECTION ( 'NONE',  ( -1.000000000000000000, -0.000000000000000000, -0.000000000000000000 ) ) ;
#11131=DIRECTION ( 'NONE',  ( -0.000000000000000000, -1.000000000000000000, -0.000000000000000000 ) ) ;
#11141=CARTESIAN_POINT ( 'NONE',  ( 45.60964950616533287, 0.000000000000000000, -15.50984893380129392 ) ) ;
#11158=ORIENTED_EDGE ( 'NONE', *, *, #8102, .T. ) ;
#11160=DIRECTION ( 'NONE',  ( -0.000000000000000000, -1.000000000000000000, -0.000000000000000000 ) ) ;
#11164=ORIENTED_EDGE ( 'NONE', *, *, #2388, .T. ) ;
#11177=CARTESIAN_POINT ( 'NONE',  ( 6.123233995736766282E-16, 3.000000000000000000, -5.000000000000000000 ) ) ;
#11182=DIRECTION ( 'NONE',  ( -0.000000000000000000, -1.000000000000000000, -0.000000000000000000 ) ) ;
#11189=CARTESIAN_POINT ( 'NONE',  ( 48.06174015963858892, 3.000000000000000000, -3.086958956539055166 ) ) ;
#11210=EDGE_CURVE ( 'NONE', #6650, #1419, #8663, .T. ) ;
#11215=PLANE ( 'NONE',  #465 ) ;
#11227=DIRECTION ( 'NONE',  ( 0.6291930273682727615, 0.000000000000000000, -0.7772490812546181127 ) ) ;
#11228=ORIENTED_EDGE ( 'NONE', *, *, #12735, .F. ) ;
#11232=LINE ( 'NONE', #1804, #9146 ) ;
#11233=SURFACE_STYLE_FILL_AREA ( #13376 ) ;
#11244=ORIENTED_EDGE ( 'NONE', *, *, #770, .F. ) ;
#11248=VECTOR ( 'NONE', #12979, 1000.000000000000000 ) ;
#11267=CARTESIAN_POINT ( 'NONE',  ( 20.03271148078819408, 3.000000000000000000, -5.075121771833452478 ) ) ;
#11279=ORIENTED_EDGE ( 'NONE', *, *, #5536, .T. ) ;
#11288=EDGE_CURVE ( 'NONE', #11648, #12786, #9339, .T. ) ;
#11296=EDGE_LOOP ( 'NONE', ( #5059, #10340, #11741, #10041 ) ) ;
#11351=CARTESIAN_POINT ( 'NONE',  ( 22.00000000000000000, 3.000000000000000000, 1.500000000000000666 ) ) ;
#11398=CARTESIAN_POINT ( 'NONE',  ( 45.22938609343211880, 0.000000000000000000, -15.43472716196784233 ) ) ;
#11411=DIRECTION ( 'NONE',  ( 0.6291930273683257191, 0.000000000000000000, -0.7772490812545752581 ) ) ;
#11429=ORIENTED_EDGE ( 'NONE', *, *, #13521, .F. ) ;
#11451=CARTESIAN_POINT ( 'NONE',  ( 41.29994854050690378, 3.000000000000000000, -5.141175130212632283 ) ) ;
#11454=CARTESIAN_POINT ( 'NONE',  ( 23.99887587215152607, 0.000000000000000000, 4.000000000000000000 ) ) ;
#11463=AXIS2_PLACEMENT_3D ( 'NONE', #8311, #4383, #3079 ) ;
#11472=VECTOR ( 'NONE', #3671, 1000.000000000000114 ) ;
#11475=EDGE_CURVE ( 'NONE', #7781, #11595, #9756, .T. ) ;
#11480=AXIS2_PLACEMENT_3D ( 'NONE', #10701, #9657, #9596 ) ;
#11490=CARTESIAN_POINT ( 'NONE',  ( 49.72134184781355515, 3.000000000000000000, -3.261665100124877981 ) ) ;
#11539=ORIENTED_EDGE ( 'NONE', *, *, #3657, .F. ) ;
#11552=DIRECTION ( 'NONE',  ( 0.000000000000000000, 0.000000000000000000, -1.000000000000000000 ) ) ;
#11570=CARTESIAN_POINT ( 'NONE',  ( 51.41686768994642165, 0.000000000000000000, -11.86457109001525545 ) ) ;
#11573=CARTESIAN_POINT ( 'NONE',  ( 41.29994854050690378, 3.000000000000000000, -6.141175130212632283 ) ) ;
#11587=VERTEX_POINT ( 'NONE', #7961 ) ;
#11588=DIRECTION ( 'NONE',  ( -0.000000000000000000, -1.000000000000000000, -0.000000000000000000 ) ) ;
#11595=VERTEX_POINT ( 'NONE', #6787 ) ;
#11598=CARTESIAN_POINT ( 'NONE',  ( 46.02418392430381999, 0.000000000000000000, -15.41988256844266658 ) ) ;
#11599=DIRECTION ( 'NONE',  ( -0.000000000000000000, -1.000000000000000000, -0.000000000000000000 ) ) ;
#11614=FACE_OUTER_BOUND ( 'NONE', #5396, .T. ) ;
#11616=VERTEX_POINT ( 'NONE', #7822 ) ;
#11630=PLANE ( 'NONE',  #12463 ) ;
#11646=FACE_OUTER_BOUND ( 'NONE', #10037, .T. ) ;
#11648=VERTEX_POINT ( 'NONE', #4735 ) ;
#11649=ORIENTED_EDGE ( 'NONE', *, *, #7355, .T. ) ;
#11658=VECTOR ( 'NONE', #12446, 1000.000000000000000 ) ;
#11686=CARTESIAN_POINT ( 'NONE',  ( 47.14458624375820506, 0.000000000000000000, -3.829406728833672613 ) ) ;
#11692=CARTESIAN_POINT ( 'NONE',  ( 49.72134184781355515, 0.000000000000000000, -3.261665100124877981 ) ) ;
#11717=AXIS2_PLACEMENT_3D ( 'NONE', #9724, #6629, #10832 ) ;
#11727=AXIS2_PLACEMENT_3D ( 'NONE', #12318, #10243, #13349 ) ;
#11741=ORIENTED_EDGE ( 'NONE', *, *, #11927, .F. ) ;
#11757=AXIS2_PLACEMENT_3D ( 'NONE', #4810, #10107, #7899 ) ;
#11762=DIRECTION ( 'NONE',  ( -0.7772490812545725936, 0.000000000000000000, -0.6291930273683289387 ) ) ;
#11767=CARTESIAN_POINT ( 'NONE',  ( 51.38094353598858532, 3.000000000000000000, -3.436371243710653722 ) ) ;
#11775=VECTOR ( 'NONE', #2458, 1000.000000000000227 ) ;
#11777=CARTESIAN_POINT ( 'NONE',  ( 45.60964950616533287, 3.000000000000000000, -14.50984893380129392 ) ) ;
#11779=DIRECTION ( 'NONE',  ( 0.000000000000000000, 0.000000000000000000, -1.000000000000000000 ) ) ;
#11784=( GEOMETRIC_REPRESENTATION_CONTEXT ( 3 ) GLOBAL_UNCERTAINTY_ASSIGNED_CONTEXT ( ( #13157 ) ) GLOBAL_UNIT_ASSIGNED_CONTEXT ( ( #835, #3712, #13440 ) ) REPRESENTATION_CONTEXT ( 'NONE', 'WORKASPACE' ) );
#11797=DIRECTION ( 'NONE',  ( -0.000000000000000000, -1.000000000000000000, 0.000000000000000000 ) ) ;
#11802=ORIENTED_EDGE ( 'NONE', *, *, #4817, .T. ) ;
#11815=CARTESIAN_POINT ( 'NONE',  ( 53.78299299645824050, 3.000000000000000000, -4.528231303176834643 ) ) ;
#11860=LINE ( 'NONE', #8543, #1770 ) ;
#11869=ORIENTED_EDGE ( 'NONE', *, *, #10044, .T. ) ;
#11882=ORIENTED_EDGE ( 'NONE', *, *, #7094, .F. ) ;
#11896=ADVANCED_FACE ( 'NONE', ( #8689 ), #7724, .F. ) ;
#11897=DIRECTION ( 'NONE',  ( 0.000000000000000000, 0.000000000000000000, -1.000000000000000000 ) ) ;
#11903=CIRCLE ( 'NONE', #11463, 1.500000000000000222 ) ;
#11916=CARTESIAN_POINT ( 'NONE',  ( 51.41686768994642165, 3.000000000000000000, -11.86457109001525545 ) ) ;
#11927=EDGE_CURVE ( 'NONE', #1592, #12572, #12012, .T. ) ;
#11945=VECTOR ( 'NONE', #12037, 1000.000000000000000 ) ;
#11967=LINE ( 'NONE', #8389, #11945 ) ;
#11972=VECTOR ( 'NONE', #2531, 1000.000000000000000 ) ;
#11973=CARTESIAN_POINT ( 'NONE',  ( 51.83140210808490167, 3.000000000000000000, -12.77460472465662988 ) ) ;
#11980=ORIENTED_EDGE ( 'NONE', *, *, #5758, .T. ) ;
#11995=EDGE_LOOP ( 'NONE', ( #1313, #1187, #2804, #13093 ) ) ;
#12012=LINE ( 'NONE', #2293, #10451 ) ;
#12014=CARTESIAN_POINT ( 'NONE',  ( 29.39270799701850123, 0.000000000000000000, -0.3930766723116408401 ) ) ;
#12024=CARTESIAN_POINT ( 'NONE',  ( 51.38094353598858532, 3.000000000000000000, -3.436371243710653722 ) ) ;
#12037=DIRECTION ( 'NONE',  ( 1.000000000000000000, 0.000000000000000000, 0.000000000000000000 ) ) ;
#12048=PLANE ( 'NONE',  #1161 ) ;
#12049=ORIENTED_EDGE ( 'NONE', *, *, #5240, .T. ) ;
#12050=PLANE ( 'NONE',  #8123 ) ;
#12066=VERTEX_POINT ( 'NONE', #12622 ) ;
#12073=PLANE ( 'NONE',  #13513 ) ;
#12074=DIRECTION ( 'NONE',  ( 0.6291930273683257191, 0.000000000000000000, -0.7772490812545752581 ) ) ;
#12090=DIRECTION ( 'NONE',  ( 0.000000000000000000, 0.000000000000000000, -1.000000000000000000 ) ) ;
#12129=EDGE_LOOP ( 'NONE', ( #11164, #847, #5597, #8652 ) ) ;
#12135=AXIS2_PLACEMENT_3D ( 'NONE', #10449, #10579, #12588 ) ;
#12146=VECTOR ( 'NONE', #2691, 1000.000000000000000 ) ;
#12157=VECTOR ( 'NONE', #5269, 1000.000000000000000 ) ;
#12169=VECTOR ( 'NONE', #223, 1000.000000000000000 ) ;
#12172=AXIS2_PLACEMENT_3D ( 'NONE', #6563, #10762, #1325 ) ;
#12187=EDGE_CURVE ( 'NONE', #1383, #13316, #2009, .T. ) ;
#12194=DIRECTION ( 'NONE',  ( -0.000000000000000000, -1.000000000000000000, -0.000000000000000000 ) ) ;
#12205=VERTEX_POINT ( 'NONE', #4136 ) ;
#12220=EDGE_LOOP ( 'NONE', ( #6447, #6295, #10432, #11649 ) ) ;
#12223=ORIENTED_EDGE ( 'NONE', *, *, #1041, .F. ) ;
#12239=ADVANCED_FACE ( 'NONE', ( #217 ), #2476, .T. ) ;
#12256=DIRECTION ( 'NONE',  ( 0.3802634127332067404, -0.000000000000000000, 0.9248782281665489657 ) ) ;
#12259=LINE ( 'NONE', #876, #7742 ) ;
#12260=ORIENTED_EDGE ( 'NONE', *, *, #4580, .F. ) ;
#12270=LINE ( 'NONE', #10046, #3091 ) ;
#12271=ADVANCED_FACE ( 'NONE', ( #11646 ), #4607, .T. ) ;
#12272=CARTESIAN_POINT ( 'NONE',  ( 45.60964950616533287, 0.000000000000000000, -14.50984893380129392 ) ) ;
#12280=CARTESIAN_POINT ( 'NONE',  ( 28.56494132578241008, 3.000000000000000000, -0.9541491613812155270 ) ) ;
#12296=ORIENTED_EDGE ( 'NONE', *, *, #7504, .F. ) ;
#12318=CARTESIAN_POINT ( 'NONE',  ( 19.65244806805498357, 3.000000000000000000, -6.000000000000000000 ) ) ;
#12335=DIRECTION ( 'NONE',  ( -0.7772490812545754801, 0.000000000000000000, -0.6291930273683253860 ) ) ;
#12345=PRODUCT_DEFINITION_CONTEXT ( 'detailed design', #7231, 'design' ) ;
#12346=VERTEX_POINT ( 'NONE', #2751 ) ;
#12364=ORIENTED_EDGE ( 'NONE', *, *, #7078, .F. ) ;
#12387=ORIENTED_EDGE ( 'NONE', *, *, #4817, .F. ) ;
#12389=( LENGTH_UNIT ( ) NAMED_UNIT ( * ) SI_UNIT ( .MILLI., .METRE. ) );
#12413=LINE ( 'NONE', #9074, #6423 ) ;
#12414=LINE ( 'NONE', #5223, #8900 ) ;
#12428=SHAPE_REPRESENTATION_RELATIONSHIP ( 'NONE' , 'NONE' ,  #8539, #13452 ) ;
#12446=DIRECTION ( 'NONE',  ( -0.000000000000000000, -1.000000000000000000, -0.000000000000000000 ) ) ;
#12459=ORIENTED_EDGE ( 'NONE', *, *, #9844, .F. ) ;
#12463=AXIS2_PLACEMENT_3D ( 'NONE', #11767, #9487, #143 ) ;
#12474=DIRECTION ( 'NONE',  ( 0.000000000000000000, 1.000000000000000000, 0.000000000000000000 ) ) ;
#12483=LINE ( 'NONE', #11573, #1007 ) ;
#12489=EDGE_CURVE ( 'NONE', #12572, #5689, #12414, .T. ) ;
#12501=LINE ( 'NONE', #5182, #731 ) ;
#12521=EDGE_CURVE ( 'NONE', #344, #2254, #12483, .T. ) ;
#12526=DIRECTION ( 'NONE',  ( 0.000000000000000000, 1.000000000000000000, 0.000000000000000000 ) ) ;
#12527=ADVANCED_FACE ( 'NONE', ( #5161 ), #9365, .T. ) ;
#12533=EDGE_CURVE ( 'NONE', #7268, #2335, #9625, .T. ) ;
#12572=VERTEX_POINT ( 'NONE', #10730 ) ;
#12575=ADVANCED_FACE ( 'NONE', ( #8513 ), #11630, .F. ) ;
#12576=AXIS2_PLACEMENT_3D ( 'NONE', #8375, #12795, #5352 ) ;
#12577=EDGE_LOOP ( 'NONE', ( #5935, #7383, #5748, #8489 ) ) ;
#12586=CARTESIAN_POINT ( 'NONE',  ( 0.000000000000000000, 0.000000000000000000, 0.000000000000000000 ) ) ;
#12588=DIRECTION ( 'NONE',  ( -0.9254744032703046130, 0.000000000000000000, -0.3788101488760216018 ) ) ;
#12591=ORIENTED_EDGE ( 'NONE', *, *, #8848, .T. ) ;
#12595=CARTESIAN_POINT ( 'NONE',  ( 22.00000000000000000, 0.000000000000000000, 0.000000000000000000 ) ) ;
#12597=CARTESIAN_POINT ( 'NONE',  ( 0.000000000000000000, 3.000000000000000000, 5.000000000000000000 ) ) ;
#12605=EDGE_CURVE ( 'NONE', #2976, #2335, #7630, .T. ) ;
#12617=AXIS2_PLACEMENT_3D ( 'NONE', #12595, #12474, #7220 ) ;
#12622=CARTESIAN_POINT ( 'NONE',  ( 46.02418392430381999, 3.000000000000000000, -15.41988256844266836 ) ) ;
#12635=CARTESIAN_POINT ( 'NONE',  ( 54.70014691233865989, 3.000000000000000000, -3.785783530882224746 ) ) ;
#12694=ORIENTED_EDGE ( 'NONE', *, *, #885, .T. ) ;
#12721=EDGE_CURVE ( 'NONE', #1968, #1592, #5583, .T. ) ;
#12735=EDGE_CURVE ( 'NONE', #12863, #12205, #10095, .T. ) ;
#12786=VERTEX_POINT ( 'NONE', #11141 ) ;
#12791=VECTOR ( 'NONE', #1352, 1000.000000000000000 ) ;
#12795=DIRECTION ( 'NONE',  ( -0.000000000000000000, -1.000000000000000000, -0.000000000000000000 ) ) ;
#12838=DIRECTION ( 'NONE',  ( 0.6291930273683233876, 0.000000000000000000, -0.7772490812545771455 ) ) ;
#12842=ORIENTED_EDGE ( 'NONE', *, *, #5758, .F. ) ;
#12854=DIRECTION ( 'NONE',  ( -0.7772490812546168915, 0.000000000000000000, -0.6291930273682743158 ) ) ;
#12861=VECTOR ( 'NONE', #3964, 1000.000000000000000 ) ;
#12863=VERTEX_POINT ( 'NONE', #11351 ) ;
#12869=STYLED_ITEM('',(#13656),#13099);
#12875=VERTEX_POINT ( 'NONE', #8302 ) ;
#12881=ADVANCED_FACE ( 'NONE', ( #8103 ), #2864, .F. ) ;
#12883=( GEOMETRIC_REPRESENTATION_CONTEXT ( 3 ) GLOBAL_UNCERTAINTY_ASSIGNED_CONTEXT ( ( #4059 ) ) GLOBAL_UNIT_ASSIGNED_CONTEXT ( ( #5864, #10062, #13232 ) ) REPRESENTATION_CONTEXT ( 'NONE', 'WORKASPACE' ) );
#12896=EDGE_CURVE ( 'NONE', #13143, #2239, #5071, .T. ) ;
#12911=ORIENTED_EDGE ( 'NONE', *, *, #7355, .F. ) ;
#12913=ORIENTED_EDGE ( 'NONE', *, *, #6838, .F. ) ;
#12916=EDGE_CURVE ( 'NONE', #1383, #11595, #944, .T. ) ;
#12922=EDGE_LOOP ( 'NONE', ( #2505, #7928, #10253, #13224 ) ) ;
#12952=ORIENTED_EDGE ( 'NONE', *, *, #6794, .T. ) ;
#12961=CARTESIAN_POINT ( 'NONE',  ( 24.82664254338761722, 0.000000000000000000, 4.561072489069574409 ) ) ;
#12965=ADVANCED_FACE ( 'NONE', ( #10923 ), #530, .F. ) ;
#12979=DIRECTION ( 'NONE',  ( -0.000000000000000000, -1.000000000000000000, -0.000000000000000000 ) ) ;
#12984=ADVANCED_FACE ( 'NONE', ( #5619 ), #4652, .F. ) ;
#12998=CARTESIAN_POINT ( 'NONE',  ( 22.00000000000000000, 3.000000000000000000, 1.500000000000000666 ) ) ;
#13043=EDGE_CURVE ( 'NONE', #344, #10535, #5158, .T. ) ;
#13044=DIRECTION ( 'NONE',  ( -0.000000000000000000, -1.000000000000000000, 0.000000000000000000 ) ) ;
#13058=ORIENTED_EDGE ( 'NONE', *, *, #3579, .F. ) ;
#13063=EDGE_CURVE ( 'NONE', #12786, #6748, #6914, .T. ) ;
#13070=AXIS2_PLACEMENT_3D ( 'NONE', #10034, #4798, #9959 ) ;
#13076=ORIENTED_EDGE ( 'NONE', *, *, #3217, .F. ) ;
#13077=ORIENTED_EDGE ( 'NONE', *, *, #11475, .T. ) ;
#13093=ORIENTED_EDGE ( 'NONE', *, *, #362, .T. ) ;
#13099=MANIFOLD_SOLID_BREP ( 'Boss-Extrude1', #13250 ) ;
#13119=LINE ( 'NONE', #799, #2268 ) ;
#13130=CARTESIAN_POINT ( 'NONE',  ( 54.70014691233865989, 0.000000000000000000, -3.785783530882224746 ) ) ;
#13143=VERTEX_POINT ( 'NONE', #1973 ) ;
#13156=ORIENTED_EDGE ( 'NONE', *, *, #4144, .T. ) ;
#13157=UNCERTAINTY_MEASURE_WITH_UNIT (LENGTH_MEASURE( 1.000000000000000082E-05 ), #835, 'distance_accuracy_value', 'NONE');
#13172=DIRECTION ( 'NONE',  ( 0.000000000000000000, -0.000000000000000000, -1.000000000000000000 ) ) ;
#13173=ORIENTED_EDGE ( 'NONE', *, *, #2431, .F. ) ;
#13203=ORIENTED_EDGE ( 'NONE', *, *, #9512, .T. ) ;
#13206=VECTOR ( 'NONE', #11124, 1000.000000000000000 ) ;
#13222=ORIENTED_EDGE ( 'NONE', *, *, #9540, .F. ) ;
#13224=ORIENTED_EDGE ( 'NONE', *, *, #7510, .F. ) ;
#13232=( NAMED_UNIT ( * ) SI_UNIT ( $, .STERADIAN. ) SOLID_ANGLE_UNIT ( ) );
#13245=CARTESIAN_POINT ( 'NONE',  ( 54.70014691233865989, 3.000000000000000000, -3.785783530882224746 ) ) ;
#13247=ORIENTED_EDGE ( 'NONE', *, *, #7014, .T. ) ;
#13250=CLOSED_SHELL ( 'NONE', ( #6000, #10575, #6392, #13523, #3120, #8202, #12984, #8097, #6413, #6324, #4501, #10296, #8416, #4430, #11896, #12575, #5403, #9697, #9111, #9607, #10815, #12271, #12881, #250, #6248, #9938, #12965, #12527, #1297, #12239, #8961, #10455, #5344 ) ) ;
#13288=LINE ( 'NONE', #10254, #9221 ) ;
#13309=DIRECTION ( 'NONE',  ( 0.000000000000000000, 0.000000000000000000, -1.000000000000000000 ) ) ;
#13310=FILL_AREA_STYLE_COLOUR ( '', #6707 ) ;
#13316=VERTEX_POINT ( 'NONE', #12024 ) ;
#13325=DIRECTION ( 'NONE',  ( -0.000000000000000000, -1.000000000000000000, -0.000000000000000000 ) ) ;
#13330=VECTOR ( 'NONE', #6589, 1000.000000000000000 ) ;
#13335=DIRECTION ( 'NONE',  ( 0.7772490812545796990, 0.000000000000000000, 0.6291930273683203900 ) ) ;
#13346=VERTEX_POINT ( 'NONE', #10973 ) ;
#13349=DIRECTION ( 'NONE',  ( 0.000000000000000000, 0.000000000000000000, -1.000000000000000000 ) ) ;
#13358=ORIENTED_EDGE ( 'NONE', *, *, #9849, .T. ) ;
#13376=FILL_AREA_STYLE ('',( #13310 ) ) ;
#13386=LINE ( 'NONE', #3933, #8186 ) ;
#13406=EDGE_CURVE ( 'NONE', #11587, #13346, #2518, .T. ) ;
#13415=VERTEX_POINT ( 'NONE', #794 ) ;
#13440=( NAMED_UNIT ( * ) SI_UNIT ( $, .STERADIAN. ) SOLID_ANGLE_UNIT ( ) );
#13452=ADVANCED_BREP_SHAPE_REPRESENTATION ( '', ( #13099, #10007 ), #12883 ) ;
#13454=ORIENTED_EDGE ( 'NONE', *, *, #7014, .F. ) ;
#13479=CYLINDRICAL_SURFACE ( 'NONE', #3980, 1.000000000000000000 ) ;
#13506=EDGE_LOOP ( 'NONE', ( #11279, #13076, #10531, #5579 ) ) ;
#13513=AXIS2_PLACEMENT_3D ( 'NONE', #572, #8953, #5716 ) ;
#13519=ORIENTED_EDGE ( 'NONE', *, *, #11210, .T. ) ;
#13521=EDGE_CURVE ( 'NONE', #12863, #6179, #782, .T. ) ;
#13523=ADVANCED_FACE ( 'NONE', ( #1052 ), #10494, .F. ) ;
#13550=FACE_OUTER_BOUND ( 'NONE', #4907, .T. ) ;
#13557=EDGE_LOOP ( 'NONE', ( #446, #7390, #3660, #12913 ) ) ;
#13563=CARTESIAN_POINT ( 'NONE',  ( 22.00000000000000000, 3.000000000000000000, 0.000000000000000000 ) ) ;
#13566=CARTESIAN_POINT ( 'NONE',  ( 0.000000000000000000, 3.000000000000000000, 0.000000000000000000 ) ) ;
#13571=CARTESIAN_POINT ( 'NONE',  ( 52.34174591811297717, 0.000000000000000000, -12.24483450274845531 ) ) ;
#13590=LINE ( 'NONE', #6018, #2520 ) ;
#13650=COLOUR_RGB('Black',0.12,0.14,0.17);
#13651=FILL_AREA_STYLE_COLOUR('',#13650);
#13652=FILL_AREA_STYLE('',(#13651));
#13653=SURFACE_STYLE_FILL_AREA(#13652);
#13654=SURFACE_SIDE_STYLE('',(#13653));
#13655=SURFACE_STYLE_USAGE(.BOTH.,#13654);
#13656=PRESENTATION_STYLE_ASSIGNMENT((#13655));
ENDSEC;
END-ISO-10303-21;
